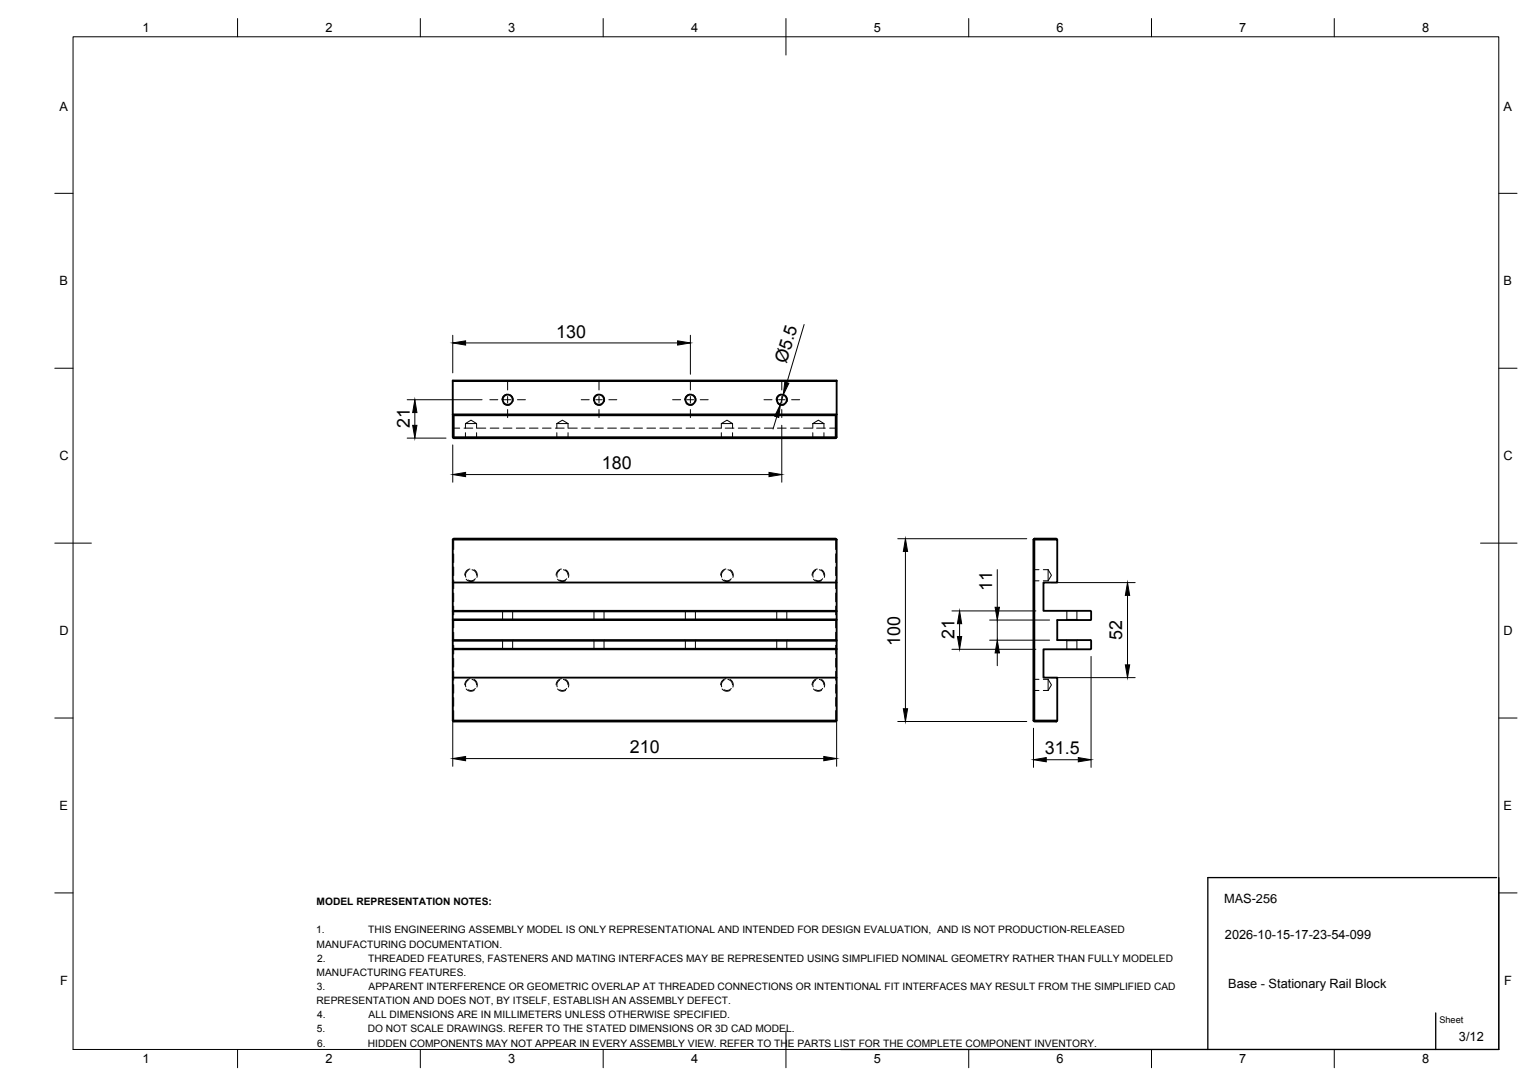
ISO-10303-21;
HEADER;
/* Generated by software containing ST-Developer
 * from STEP Tools, Inc. (www.steptools.com) 
 */

FILE_DESCRIPTION(
/* description */ (''),
/* implementation_level */ '2;1');

FILE_NAME(
/* name */ 'Base - Stationary Rail Block.step',
/* time_stamp */ '2026-10-14T18:40:07-07:00',
/* author */ (''),
/* organization */ (''),
/* preprocessor_version */ 'ST-DEVELOPER v20.2',
/* originating_system */ 'Autodesk Translation Framework v15.15.0.0',
/* authorisation */ '');

FILE_SCHEMA (('AUTOMOTIVE_DESIGN { 1 0 10303 214 3 1 1 }'));
ENDSEC;

DATA;
#10=MECHANICAL_DESIGN_GEOMETRIC_PRESENTATION_REPRESENTATION('',(#831),#81040);
#811=SHAPE_REPRESENTATION_RELATIONSHIP('SRR','None',#81130,#821);
#821=ADVANCED_BREP_SHAPE_REPRESENTATION('',(#841),#81030);
#831=STYLED_ITEM('',(#81189),#841);
#841=MANIFOLD_SOLID_BREP('Body1',#15084);
#851=CYLINDRICAL_SURFACE('',#15214,2.74999999999999);
#852=CYLINDRICAL_SURFACE('',#15218,2.75);
#853=CYLINDRICAL_SURFACE('',#15222,2.75);
#854=CYLINDRICAL_SURFACE('',#15226,2.75);
#855=CYLINDRICAL_SURFACE('',#15235,2.74999999999999);
#856=CYLINDRICAL_SURFACE('',#15239,2.75);
#857=CYLINDRICAL_SURFACE('',#15243,2.75);
#858=CYLINDRICAL_SURFACE('',#15247,2.75);
#859=CYLINDRICAL_SURFACE('',#15260,3.05);
#860=CYLINDRICAL_SURFACE('',#15264,3.05);
#861=CYLINDRICAL_SURFACE('',#15268,3.05);
#862=CYLINDRICAL_SURFACE('',#15272,3.05);
#863=CYLINDRICAL_SURFACE('',#15276,3.05);
#864=CYLINDRICAL_SURFACE('',#15280,3.05);
#865=CYLINDRICAL_SURFACE('',#15284,3.05);
#866=CYLINDRICAL_SURFACE('',#15288,3.05);
#1083=FACE_BOUND('',#2351,.T.);
#1084=FACE_BOUND('',#2352,.T.);
#1085=FACE_BOUND('',#2353,.T.);
#1086=FACE_BOUND('',#2354,.T.);
#1087=FACE_BOUND('',#2364,.T.);
#1088=FACE_BOUND('',#2365,.T.);
#1089=FACE_BOUND('',#2366,.T.);
#1090=FACE_BOUND('',#2367,.T.);
#1091=FACE_BOUND('',#2377,.T.);
#1092=FACE_BOUND('',#2378,.T.);
#1093=FACE_BOUND('',#2379,.T.);
#1094=FACE_BOUND('',#2380,.T.);
#1095=FACE_BOUND('',#2381,.T.);
#1096=FACE_BOUND('',#2382,.T.);
#1097=FACE_BOUND('',#2383,.T.);
#1098=FACE_BOUND('',#2384,.T.);
#1099=FACE_BOUND('',#2427,.T.);
#1100=FACE_BOUND('',#2428,.T.);
#1101=FACE_BOUND('',#2429,.T.);
#1102=FACE_BOUND('',#2430,.T.);
#1103=FACE_BOUND('',#2439,.T.);
#1104=FACE_BOUND('',#2440,.T.);
#1105=FACE_BOUND('',#2441,.T.);
#1106=FACE_BOUND('',#2442,.T.);
#1211=PLANE('',#15210);
#1212=PLANE('',#15231);
#1213=PLANE('',#15252);
#1214=PLANE('',#15298);
#1215=PLANE('',#15299);
#1216=PLANE('',#15300);
#1217=PLANE('',#15301);
#1218=PLANE('',#15302);
#1219=PLANE('',#15303);
#1220=PLANE('',#15304);
#1221=PLANE('',#15305);
#1222=PLANE('',#15306);
#1223=PLANE('',#15307);
#1224=PLANE('',#15308);
#1225=PLANE('',#15309);
#1226=PLANE('',#15310);
#1227=PLANE('',#15311);
#1228=PLANE('',#15312);
#1229=PLANE('',#15313);
#1230=PLANE('',#15314);
#1231=PLANE('',#15315);
#1232=PLANE('',#15316);
#1233=PLANE('',#15317);
#1234=PLANE('',#15318);
#1235=PLANE('',#15319);
#1236=PLANE('',#15320);
#1237=PLANE('',#15321);
#1238=PLANE('',#15322);
#1239=PLANE('',#15323);
#1240=PLANE('',#15324);
#1241=PLANE('',#15325);
#1242=PLANE('',#15326);
#1606=FACE_OUTER_BOUND('',#2349,.T.);
#1607=FACE_OUTER_BOUND('',#2350,.T.);
#1608=FACE_OUTER_BOUND('',#2355,.T.);
#1609=FACE_OUTER_BOUND('',#2356,.T.);
#1610=FACE_OUTER_BOUND('',#2357,.T.);
#1611=FACE_OUTER_BOUND('',#2358,.T.);
#1612=FACE_OUTER_BOUND('',#2359,.T.);
#1613=FACE_OUTER_BOUND('',#2360,.T.);
#1614=FACE_OUTER_BOUND('',#2361,.T.);
#1615=FACE_OUTER_BOUND('',#2362,.T.);
#1616=FACE_OUTER_BOUND('',#2363,.T.);
#1617=FACE_OUTER_BOUND('',#2368,.T.);
#1618=FACE_OUTER_BOUND('',#2369,.T.);
#1619=FACE_OUTER_BOUND('',#2370,.T.);
#1620=FACE_OUTER_BOUND('',#2371,.T.);
#1621=FACE_OUTER_BOUND('',#2372,.T.);
#1622=FACE_OUTER_BOUND('',#2373,.T.);
#1623=FACE_OUTER_BOUND('',#2374,.T.);
#1624=FACE_OUTER_BOUND('',#2375,.T.);
#1625=FACE_OUTER_BOUND('',#2376,.T.);
#1626=FACE_OUTER_BOUND('',#2385,.T.);
#1627=FACE_OUTER_BOUND('',#2386,.T.);
#1628=FACE_OUTER_BOUND('',#2387,.T.);
#1629=FACE_OUTER_BOUND('',#2388,.T.);
#1630=FACE_OUTER_BOUND('',#2389,.T.);
#1631=FACE_OUTER_BOUND('',#2390,.T.);
#1632=FACE_OUTER_BOUND('',#2391,.T.);
#1633=FACE_OUTER_BOUND('',#2392,.T.);
#1634=FACE_OUTER_BOUND('',#2393,.T.);
#1635=FACE_OUTER_BOUND('',#2394,.T.);
#1636=FACE_OUTER_BOUND('',#2395,.T.);
#1637=FACE_OUTER_BOUND('',#2396,.T.);
#1638=FACE_OUTER_BOUND('',#2397,.T.);
#1639=FACE_OUTER_BOUND('',#2398,.T.);
#1640=FACE_OUTER_BOUND('',#2399,.T.);
#1641=FACE_OUTER_BOUND('',#2400,.T.);
#1642=FACE_OUTER_BOUND('',#2401,.T.);
#1643=FACE_OUTER_BOUND('',#2402,.T.);
#1644=FACE_OUTER_BOUND('',#2403,.T.);
#1645=FACE_OUTER_BOUND('',#2404,.T.);
#1646=FACE_OUTER_BOUND('',#2405,.T.);
#1647=FACE_OUTER_BOUND('',#2406,.T.);
#1648=FACE_OUTER_BOUND('',#2407,.T.);
#1649=FACE_OUTER_BOUND('',#2408,.T.);
#1650=FACE_OUTER_BOUND('',#2409,.T.);
#1651=FACE_OUTER_BOUND('',#2410,.T.);
#1652=FACE_OUTER_BOUND('',#2411,.T.);
#1653=FACE_OUTER_BOUND('',#2412,.T.);
#1654=FACE_OUTER_BOUND('',#2413,.T.);
#1655=FACE_OUTER_BOUND('',#2414,.T.);
#1656=FACE_OUTER_BOUND('',#2415,.T.);
#1657=FACE_OUTER_BOUND('',#2416,.T.);
#1658=FACE_OUTER_BOUND('',#2417,.T.);
#1659=FACE_OUTER_BOUND('',#2418,.T.);
#1660=FACE_OUTER_BOUND('',#2419,.T.);
#1661=FACE_OUTER_BOUND('',#2420,.T.);
#1662=FACE_OUTER_BOUND('',#2421,.T.);
#1663=FACE_OUTER_BOUND('',#2422,.T.);
#1664=FACE_OUTER_BOUND('',#2423,.T.);
#1665=FACE_OUTER_BOUND('',#2424,.T.);
#1666=FACE_OUTER_BOUND('',#2425,.T.);
#1667=FACE_OUTER_BOUND('',#2426,.T.);
#1668=FACE_OUTER_BOUND('',#2431,.T.);
#1669=FACE_OUTER_BOUND('',#2432,.T.);
#1670=FACE_OUTER_BOUND('',#2433,.T.);
#1671=FACE_OUTER_BOUND('',#2434,.T.);
#1672=FACE_OUTER_BOUND('',#2435,.T.);
#1673=FACE_OUTER_BOUND('',#2436,.T.);
#1674=FACE_OUTER_BOUND('',#2437,.T.);
#1675=FACE_OUTER_BOUND('',#2438,.T.);
#1676=FACE_OUTER_BOUND('',#2443,.T.);
#1677=FACE_OUTER_BOUND('',#2444,.T.);
#2349=EDGE_LOOP('',(#9782,#9783,#9784,#9785));
#2350=EDGE_LOOP('',(#9786,#9787,#9788,#9789));
#2351=EDGE_LOOP('',(#9790));
#2352=EDGE_LOOP('',(#9791));
#2353=EDGE_LOOP('',(#9792));
#2354=EDGE_LOOP('',(#9793));
#2355=EDGE_LOOP('',(#9794,#9795,#9796,#9797));
#2356=EDGE_LOOP('',(#9798,#9799,#9800,#9801));
#2357=EDGE_LOOP('',(#9802,#9803,#9804,#9805));
#2358=EDGE_LOOP('',(#9806,#9807,#9808,#9809));
#2359=EDGE_LOOP('',(#9810,#9811,#9812,#9813));
#2360=EDGE_LOOP('',(#9814,#9815,#9816,#9817));
#2361=EDGE_LOOP('',(#9818,#9819,#9820,#9821));
#2362=EDGE_LOOP('',(#9822,#9823,#9824,#9825));
#2363=EDGE_LOOP('',(#9826,#9827,#9828,#9829));
#2364=EDGE_LOOP('',(#9830));
#2365=EDGE_LOOP('',(#9831));
#2366=EDGE_LOOP('',(#9832));
#2367=EDGE_LOOP('',(#9833));
#2368=EDGE_LOOP('',(#9834,#9835,#9836,#9837));
#2369=EDGE_LOOP('',(#9838,#9839,#9840,#9841));
#2370=EDGE_LOOP('',(#9842,#9843,#9844,#9845));
#2371=EDGE_LOOP('',(#9846,#9847,#9848,#9849));
#2372=EDGE_LOOP('',(#9850,#9851,#9852,#9853));
#2373=EDGE_LOOP('',(#9854,#9855,#9856,#9857));
#2374=EDGE_LOOP('',(#9858,#9859,#9860,#9861));
#2375=EDGE_LOOP('',(#9862,#9863,#9864,#9865));
#2376=EDGE_LOOP('',(#9866,#9867,#9868,#9869));
#2377=EDGE_LOOP('',(#9870));
#2378=EDGE_LOOP('',(#9871));
#2379=EDGE_LOOP('',(#9872));
#2380=EDGE_LOOP('',(#9873));
#2381=EDGE_LOOP('',(#9874));
#2382=EDGE_LOOP('',(#9875));
#2383=EDGE_LOOP('',(#9876));
#2384=EDGE_LOOP('',(#9877));
#2385=EDGE_LOOP('',(#9878,#9879,#9880,#9881));
#2386=EDGE_LOOP('',(#9882,#9883,#9884,#9885));
#2387=EDGE_LOOP('',(#9886,#9887,#9888,#9889));
#2388=EDGE_LOOP('',(#9890,#9891,#9892,#9893));
#2389=EDGE_LOOP('',(#9894,#9895,#9896,#9897));
#2390=EDGE_LOOP('',(#9898,#9899,#9900,#9901));
#2391=EDGE_LOOP('',(#9902,#9903,#9904,#9905));
#2392=EDGE_LOOP('',(#9906,#9907,#9908,#9909));
#2393=EDGE_LOOP('',(#9910,#9911,#9912,#9913));
#2394=EDGE_LOOP('',(#9914,#9915,#9916,#9917));
#2395=EDGE_LOOP('',(#9918,#9919,#9920,#9921));
#2396=EDGE_LOOP('',(#9922,#9923,#9924,#9925));
#2397=EDGE_LOOP('',(#9926,#9927,#9928,#9929));
#2398=EDGE_LOOP('',(#9930,#9931,#9932,#9933));
#2399=EDGE_LOOP('',(#9934,#9935,#9936,#9937));
#2400=EDGE_LOOP('',(#9938,#9939,#9940));
#2401=EDGE_LOOP('',(#9941,#9942,#9943));
#2402=EDGE_LOOP('',(#9944,#9945,#9946));
#2403=EDGE_LOOP('',(#9947,#9948,#9949));
#2404=EDGE_LOOP('',(#9950,#9951,#9952));
#2405=EDGE_LOOP('',(#9953,#9954,#9955));
#2406=EDGE_LOOP('',(#9956,#9957,#9958));
#2407=EDGE_LOOP('',(#9959,#9960,#9961));
#2408=EDGE_LOOP('',(#9962,#9963,#9964,#9965,#9966));
#2409=EDGE_LOOP('',(#9967,#9968,#9969,#9970,#9971,#9972));
#2410=EDGE_LOOP('',(#9973,#9974,#9975,#9976,#9977,#9978,#9979,#9980,#9981,
#9982,#9983,#9984,#9985,#9986,#9987,#9988,#9989,#9990,#9991,#9992));
#2411=EDGE_LOOP('',(#9993,#9994,#9995,#9996));
#2412=EDGE_LOOP('',(#9997,#9998,#9999,#10000,#10001,#10002));
#2413=EDGE_LOOP('',(#10003,#10004,#10005,#10006,#10007));
#2414=EDGE_LOOP('',(#10008,#10009,#10010,#10011));
#2415=EDGE_LOOP('',(#10012,#10013,#10014,#10015,#10016));
#2416=EDGE_LOOP('',(#10017,#10018,#10019,#10020,#10021,#10022));
#2417=EDGE_LOOP('',(#10023,#10024,#10025,#10026,#10027,#10028));
#2418=EDGE_LOOP('',(#10029,#10030,#10031,#10032,#10033));
#2419=EDGE_LOOP('',(#10034,#10035,#10036,#10037,#10038,#10039,#10040,#10041,
#10042,#10043,#10044,#10045,#10046,#10047,#10048,#10049,#10050,#10051,#10052,
#10053));
#2420=EDGE_LOOP('',(#10054,#10055,#10056,#10057));
#2421=EDGE_LOOP('',(#10058,#10059,#10060,#10061));
#2422=EDGE_LOOP('',(#10062,#10063,#10064,#10065));
#2423=EDGE_LOOP('',(#10066,#10067,#10068,#10069));
#2424=EDGE_LOOP('',(#10070,#10071,#10072,#10073));
#2425=EDGE_LOOP('',(#10074,#10075,#10076,#10077));
#2426=EDGE_LOOP('',(#10078,#10079,#10080,#10081));
#2427=EDGE_LOOP('',(#10082));
#2428=EDGE_LOOP('',(#10083));
#2429=EDGE_LOOP('',(#10084));
#2430=EDGE_LOOP('',(#10085));
#2431=EDGE_LOOP('',(#10086,#10087,#10088,#10089));
#2432=EDGE_LOOP('',(#10090,#10091,#10092,#10093));
#2433=EDGE_LOOP('',(#10094,#10095,#10096,#10097));
#2434=EDGE_LOOP('',(#10098,#10099,#10100,#10101));
#2435=EDGE_LOOP('',(#10102,#10103,#10104,#10105));
#2436=EDGE_LOOP('',(#10106,#10107,#10108,#10109));
#2437=EDGE_LOOP('',(#10110,#10111,#10112,#10113));
#2438=EDGE_LOOP('',(#10114,#10115,#10116,#10117));
#2439=EDGE_LOOP('',(#10118));
#2440=EDGE_LOOP('',(#10119));
#2441=EDGE_LOOP('',(#10120));
#2442=EDGE_LOOP('',(#10121));
#2443=EDGE_LOOP('',(#10122,#10123,#10124,#10125));
#2444=EDGE_LOOP('',(#10126,#10127,#10128,#10129));
#3220=LINE('',#20568,#4332);
#3221=LINE('',#20573,#4333);
#3222=LINE('',#20575,#4334);
#3223=LINE('',#20577,#4335);
#3224=LINE('',#20578,#4336);
#3225=LINE('',#20587,#4337);
#3226=LINE('',#20592,#4338);
#3227=LINE('',#20595,#4339);
#3228=LINE('',#20600,#4340);
#3229=LINE('',#20603,#4341);
#3230=LINE('',#20608,#4342);
#3231=LINE('',#20611,#4343);
#3232=LINE('',#20617,#4344);
#3233=LINE('',#20622,#4345);
#3234=LINE('',#20624,#4346);
#3235=LINE('',#20626,#4347);
#3236=LINE('',#20627,#4348);
#3237=LINE('',#20636,#4349);
#3238=LINE('',#20641,#4350);
#3239=LINE('',#20644,#4351);
#3240=LINE('',#20649,#4352);
#3241=LINE('',#20652,#4353);
#3242=LINE('',#20657,#4354);
#3243=LINE('',#20660,#4355);
#3244=LINE('',#20666,#4356);
#3245=LINE('',#20671,#4357);
#3246=LINE('',#20673,#4358);
#3247=LINE('',#20675,#4359);
#3248=LINE('',#20676,#4360);
#3249=LINE('',#20693,#4361);
#3250=LINE('',#20698,#4362);
#3251=LINE('',#20701,#4363);
#3252=LINE('',#20706,#4364);
#3253=LINE('',#20709,#4365);
#3254=LINE('',#20714,#4366);
#3255=LINE('',#20717,#4367);
#3256=LINE('',#20722,#4368);
#3257=LINE('',#20725,#4369);
#3258=LINE('',#20730,#4370);
#3259=LINE('',#20733,#4371);
#3260=LINE('',#20738,#4372);
#3261=LINE('',#20741,#4373);
#3262=LINE('',#20746,#4374);
#3263=LINE('',#20749,#4375);
#3264=LINE('',#20753,#4376);
#3265=LINE('',#20756,#4377);
#3266=LINE('',#20759,#4378);
#3267=LINE('',#20762,#4379);
#3268=LINE('',#20765,#4380);
#3269=LINE('',#20768,#4381);
#3270=LINE('',#20771,#4382);
#3271=LINE('',#20774,#4383);
#3272=LINE('',#20778,#4384);
#3273=LINE('',#20780,#4385);
#3274=LINE('',#20782,#4386);
#3275=LINE('',#20784,#4387);
#3276=LINE('',#20785,#4388);
#3277=LINE('',#20788,#4389);
#3278=LINE('',#20790,#4390);
#3279=LINE('',#20791,#4391);
#3280=LINE('',#20792,#4392);
#3281=LINE('',#20795,#4393);
#3282=LINE('',#20797,#4394);
#3283=LINE('',#20799,#4395);
#3284=LINE('',#20801,#4396);
#3285=LINE('',#20803,#4397);
#3286=LINE('',#20805,#4398);
#3287=LINE('',#20806,#4399);
#3288=LINE('',#20807,#4400);
#3289=LINE('',#20809,#4401);
#3290=LINE('',#20811,#4402);
#3291=LINE('',#20813,#4403);
#3292=LINE('',#20815,#4404);
#3293=LINE('',#20817,#4405);
#3294=LINE('',#20819,#4406);
#3295=LINE('',#20821,#4407);
#3296=LINE('',#20822,#4408);
#3297=LINE('',#20825,#4409);
#3298=LINE('',#20827,#4410);
#3299=LINE('',#20828,#4411);
#3300=LINE('',#20831,#4412);
#3301=LINE('',#20833,#4413);
#3302=LINE('',#20835,#4414);
#3303=LINE('',#20836,#4415);
#3304=LINE('',#20839,#4416);
#3305=LINE('',#20840,#4417);
#3306=LINE('',#20843,#4418);
#3307=LINE('',#20844,#4419);
#3308=LINE('',#20847,#4420);
#3309=LINE('',#20849,#4421);
#3310=LINE('',#20850,#4422);
#3311=LINE('',#20853,#4423);
#3312=LINE('',#20855,#4424);
#3313=LINE('',#20856,#4425);
#3314=LINE('',#20859,#4426);
#3315=LINE('',#20860,#4427);
#3316=LINE('',#20862,#4428);
#3317=LINE('',#20863,#4429);
#3318=LINE('',#20866,#4430);
#3319=LINE('',#20868,#4431);
#3320=LINE('',#20870,#4432);
#3321=LINE('',#20872,#4433);
#3322=LINE('',#20874,#4434);
#3323=LINE('',#20876,#4435);
#3324=LINE('',#20877,#4436);
#3325=LINE('',#20878,#4437);
#3326=LINE('',#20880,#4438);
#3327=LINE('',#20882,#4439);
#3328=LINE('',#20884,#4440);
#3329=LINE('',#20886,#4441);
#3330=LINE('',#20888,#4442);
#3331=LINE('',#20890,#4443);
#3332=LINE('',#20891,#4444);
#3333=LINE('',#20893,#4445);
#3334=LINE('',#20894,#4446);
#3335=LINE('',#20896,#4447);
#3336=LINE('',#20899,#4448);
#3337=LINE('',#20901,#4449);
#3338=LINE('',#20903,#4450);
#3339=LINE('',#20905,#4451);
#3340=LINE('',#20907,#4452);
#3341=LINE('',#20909,#4453);
#3342=LINE('',#20912,#4454);
#3343=LINE('',#20914,#4455);
#3344=LINE('',#20918,#4456);
#3345=LINE('',#20920,#4457);
#4332=VECTOR('',#16628,2.89999999999999);
#4333=VECTOR('',#16633,10.);
#4334=VECTOR('',#16634,10.);
#4335=VECTOR('',#16635,10.);
#4336=VECTOR('',#16636,10.);
#4337=VECTOR('',#16645,2.74999999999999);
#4338=VECTOR('',#16652,2.9);
#4339=VECTOR('',#16655,2.75);
#4340=VECTOR('',#16662,2.9);
#4341=VECTOR('',#16665,2.75);
#4342=VECTOR('',#16672,2.9);
#4343=VECTOR('',#16675,2.75);
#4344=VECTOR('',#16682,2.89999999999999);
#4345=VECTOR('',#16687,10.);
#4346=VECTOR('',#16688,10.);
#4347=VECTOR('',#16689,10.);
#4348=VECTOR('',#16690,10.);
#4349=VECTOR('',#16699,2.74999999999999);
#4350=VECTOR('',#16706,2.9);
#4351=VECTOR('',#16709,2.75);
#4352=VECTOR('',#16716,2.9);
#4353=VECTOR('',#16719,2.75);
#4354=VECTOR('',#16726,2.9);
#4355=VECTOR('',#16729,2.75);
#4356=VECTOR('',#16736,3.24999999999999);
#4357=VECTOR('',#16741,10.);
#4358=VECTOR('',#16742,10.);
#4359=VECTOR('',#16743,10.);
#4360=VECTOR('',#16744,10.);
#4361=VECTOR('',#16761,3.05);
#4362=VECTOR('',#16768,3.24999999999999);
#4363=VECTOR('',#16771,3.05);
#4364=VECTOR('',#16778,3.25);
#4365=VECTOR('',#16781,3.05);
#4366=VECTOR('',#16788,3.25);
#4367=VECTOR('',#16791,3.05);
#4368=VECTOR('',#16798,3.25);
#4369=VECTOR('',#16801,3.05);
#4370=VECTOR('',#16808,3.25);
#4371=VECTOR('',#16811,3.05);
#4372=VECTOR('',#16818,3.24999999999999);
#4373=VECTOR('',#16821,3.05);
#4374=VECTOR('',#16828,3.24999999999999);
#4375=VECTOR('',#16831,3.05);
#4376=VECTOR('',#16836,1.525);
#4377=VECTOR('',#16839,1.525);
#4378=VECTOR('',#16842,1.525);
#4379=VECTOR('',#16845,1.525);
#4380=VECTOR('',#16848,1.525);
#4381=VECTOR('',#16851,1.525);
#4382=VECTOR('',#16854,1.525);
#4383=VECTOR('',#16857,1.525);
#4384=VECTOR('',#16860,10.);
#4385=VECTOR('',#16861,10.);
#4386=VECTOR('',#16862,10.);
#4387=VECTOR('',#16863,10.);
#4388=VECTOR('',#16864,10.);
#4389=VECTOR('',#16867,10.);
#4390=VECTOR('',#16868,10.);
#4391=VECTOR('',#16869,10.);
#4392=VECTOR('',#16870,10.);
#4393=VECTOR('',#16873,10.);
#4394=VECTOR('',#16874,10.);
#4395=VECTOR('',#16875,10.);
#4396=VECTOR('',#16876,10.);
#4397=VECTOR('',#16877,10.);
#4398=VECTOR('',#16878,10.);
#4399=VECTOR('',#16879,10.);
#4400=VECTOR('',#16880,10.);
#4401=VECTOR('',#16881,10.);
#4402=VECTOR('',#16882,10.);
#4403=VECTOR('',#16883,10.);
#4404=VECTOR('',#16884,10.);
#4405=VECTOR('',#16885,10.);
#4406=VECTOR('',#16886,10.);
#4407=VECTOR('',#16887,10.);
#4408=VECTOR('',#16888,10.);
#4409=VECTOR('',#16891,10.);
#4410=VECTOR('',#16892,10.);
#4411=VECTOR('',#16893,10.);
#4412=VECTOR('',#16896,10.);
#4413=VECTOR('',#16897,10.);
#4414=VECTOR('',#16898,10.);
#4415=VECTOR('',#16899,10.);
#4416=VECTOR('',#16902,10.);
#4417=VECTOR('',#16903,10.);
#4418=VECTOR('',#16906,10.);
#4419=VECTOR('',#16907,10.);
#4420=VECTOR('',#16910,10.);
#4421=VECTOR('',#16911,10.);
#4422=VECTOR('',#16912,10.);
#4423=VECTOR('',#16915,10.);
#4424=VECTOR('',#16916,10.);
#4425=VECTOR('',#16917,10.);
#4426=VECTOR('',#16920,10.);
#4427=VECTOR('',#16921,10.);
#4428=VECTOR('',#16924,10.);
#4429=VECTOR('',#16925,10.);
#4430=VECTOR('',#16928,10.);
#4431=VECTOR('',#16929,10.);
#4432=VECTOR('',#16930,10.);
#4433=VECTOR('',#16931,10.);
#4434=VECTOR('',#16932,10.);
#4435=VECTOR('',#16933,10.);
#4436=VECTOR('',#16934,10.);
#4437=VECTOR('',#16935,10.);
#4438=VECTOR('',#16936,10.);
#4439=VECTOR('',#16937,10.);
#4440=VECTOR('',#16938,10.);
#4441=VECTOR('',#16939,10.);
#4442=VECTOR('',#16940,10.);
#4443=VECTOR('',#16941,10.);
#4444=VECTOR('',#16942,10.);
#4445=VECTOR('',#16945,10.);
#4446=VECTOR('',#16946,10.);
#4447=VECTOR('',#16949,10.);
#4448=VECTOR('',#16954,10.);
#4449=VECTOR('',#16957,10.);
#4450=VECTOR('',#16960,10.);
#4451=VECTOR('',#16963,10.);
#4452=VECTOR('',#16966,10.);
#4453=VECTOR('',#16969,10.);
#4454=VECTOR('',#16974,10.);
#4455=VECTOR('',#16977,10.);
#4456=VECTOR('',#16984,10.);
#4457=VECTOR('',#16987,10.);
#5444=CIRCLE('',#15208,2.74999999999999);
#5445=CIRCLE('',#15209,3.05);
#5446=CIRCLE('',#15211,3.05);
#5447=CIRCLE('',#15212,3.05);
#5448=CIRCLE('',#15213,3.05);
#5449=CIRCLE('',#15215,2.74999999999999);
#5450=CIRCLE('',#15217,2.75);
#5451=CIRCLE('',#15219,2.75);
#5452=CIRCLE('',#15221,2.75);
#5453=CIRCLE('',#15223,2.75);
#5454=CIRCLE('',#15225,2.75);
#5455=CIRCLE('',#15227,2.75);
#5456=CIRCLE('',#15229,2.74999999999999);
#5457=CIRCLE('',#15230,3.05);
#5458=CIRCLE('',#15232,3.05);
#5459=CIRCLE('',#15233,3.05);
#5460=CIRCLE('',#15234,3.05);
#5461=CIRCLE('',#15236,2.74999999999999);
#5462=CIRCLE('',#15238,2.75);
#5463=CIRCLE('',#15240,2.75);
#5464=CIRCLE('',#15242,2.75);
#5465=CIRCLE('',#15244,2.75);
#5466=CIRCLE('',#15246,2.75);
#5467=CIRCLE('',#15248,2.75);
#5468=CIRCLE('',#15250,3.05);
#5469=CIRCLE('',#15251,3.44999999999999);
#5470=CIRCLE('',#15253,3.44999999999999);
#5471=CIRCLE('',#15254,3.45);
#5472=CIRCLE('',#15255,3.45);
#5473=CIRCLE('',#15256,3.44999999999999);
#5474=CIRCLE('',#15257,3.44999999999999);
#5475=CIRCLE('',#15258,3.45);
#5476=CIRCLE('',#15259,3.45);
#5477=CIRCLE('',#15261,3.05);
#5478=CIRCLE('',#15263,3.05);
#5479=CIRCLE('',#15265,3.05);
#5480=CIRCLE('',#15267,3.05);
#5481=CIRCLE('',#15269,3.05);
#5482=CIRCLE('',#15271,3.05);
#5483=CIRCLE('',#15273,3.05);
#5484=CIRCLE('',#15275,3.05);
#5485=CIRCLE('',#15277,3.05);
#5486=CIRCLE('',#15279,3.05);
#5487=CIRCLE('',#15281,3.05);
#5488=CIRCLE('',#15283,3.05);
#5489=CIRCLE('',#15285,3.05);
#5490=CIRCLE('',#15287,3.05);
#5491=CIRCLE('',#15289,3.05);
#6021=VERTEX_POINT('',#20565);
#6022=VERTEX_POINT('',#20567);
#6023=VERTEX_POINT('',#20571);
#6024=VERTEX_POINT('',#20572);
#6025=VERTEX_POINT('',#20574);
#6026=VERTEX_POINT('',#20576);
#6027=VERTEX_POINT('',#20579);
#6028=VERTEX_POINT('',#20581);
#6029=VERTEX_POINT('',#20583);
#6030=VERTEX_POINT('',#20586);
#6031=VERTEX_POINT('',#20590);
#6032=VERTEX_POINT('',#20594);
#6033=VERTEX_POINT('',#20598);
#6034=VERTEX_POINT('',#20602);
#6035=VERTEX_POINT('',#20606);
#6036=VERTEX_POINT('',#20610);
#6037=VERTEX_POINT('',#20614);
#6038=VERTEX_POINT('',#20616);
#6039=VERTEX_POINT('',#20620);
#6040=VERTEX_POINT('',#20621);
#6041=VERTEX_POINT('',#20623);
#6042=VERTEX_POINT('',#20625);
#6043=VERTEX_POINT('',#20628);
#6044=VERTEX_POINT('',#20630);
#6045=VERTEX_POINT('',#20632);
#6046=VERTEX_POINT('',#20635);
#6047=VERTEX_POINT('',#20639);
#6048=VERTEX_POINT('',#20643);
#6049=VERTEX_POINT('',#20647);
#6050=VERTEX_POINT('',#20651);
#6051=VERTEX_POINT('',#20655);
#6052=VERTEX_POINT('',#20659);
#6053=VERTEX_POINT('',#20663);
#6054=VERTEX_POINT('',#20665);
#6055=VERTEX_POINT('',#20669);
#6056=VERTEX_POINT('',#20670);
#6057=VERTEX_POINT('',#20672);
#6058=VERTEX_POINT('',#20674);
#6059=VERTEX_POINT('',#20677);
#6060=VERTEX_POINT('',#20679);
#6061=VERTEX_POINT('',#20681);
#6062=VERTEX_POINT('',#20683);
#6063=VERTEX_POINT('',#20685);
#6064=VERTEX_POINT('',#20687);
#6065=VERTEX_POINT('',#20689);
#6066=VERTEX_POINT('',#20692);
#6067=VERTEX_POINT('',#20696);
#6068=VERTEX_POINT('',#20700);
#6069=VERTEX_POINT('',#20704);
#6070=VERTEX_POINT('',#20708);
#6071=VERTEX_POINT('',#20712);
#6072=VERTEX_POINT('',#20716);
#6073=VERTEX_POINT('',#20720);
#6074=VERTEX_POINT('',#20724);
#6075=VERTEX_POINT('',#20728);
#6076=VERTEX_POINT('',#20732);
#6077=VERTEX_POINT('',#20736);
#6078=VERTEX_POINT('',#20740);
#6079=VERTEX_POINT('',#20744);
#6080=VERTEX_POINT('',#20748);
#6081=VERTEX_POINT('',#20752);
#6082=VERTEX_POINT('',#20755);
#6083=VERTEX_POINT('',#20758);
#6084=VERTEX_POINT('',#20761);
#6085=VERTEX_POINT('',#20764);
#6086=VERTEX_POINT('',#20767);
#6087=VERTEX_POINT('',#20770);
#6088=VERTEX_POINT('',#20773);
#6089=VERTEX_POINT('',#20776);
#6090=VERTEX_POINT('',#20777);
#6091=VERTEX_POINT('',#20779);
#6092=VERTEX_POINT('',#20781);
#6093=VERTEX_POINT('',#20783);
#6094=VERTEX_POINT('',#20787);
#6095=VERTEX_POINT('',#20789);
#6096=VERTEX_POINT('',#20794);
#6097=VERTEX_POINT('',#20796);
#6098=VERTEX_POINT('',#20798);
#6099=VERTEX_POINT('',#20800);
#6100=VERTEX_POINT('',#20802);
#6101=VERTEX_POINT('',#20804);
#6102=VERTEX_POINT('',#20808);
#6103=VERTEX_POINT('',#20810);
#6104=VERTEX_POINT('',#20812);
#6105=VERTEX_POINT('',#20814);
#6106=VERTEX_POINT('',#20816);
#6107=VERTEX_POINT('',#20818);
#6108=VERTEX_POINT('',#20820);
#6109=VERTEX_POINT('',#20824);
#6110=VERTEX_POINT('',#20826);
#6111=VERTEX_POINT('',#20830);
#6112=VERTEX_POINT('',#20832);
#6113=VERTEX_POINT('',#20834);
#6114=VERTEX_POINT('',#20838);
#6115=VERTEX_POINT('',#20842);
#6116=VERTEX_POINT('',#20846);
#6117=VERTEX_POINT('',#20848);
#6118=VERTEX_POINT('',#20852);
#6119=VERTEX_POINT('',#20854);
#6120=VERTEX_POINT('',#20858);
#6121=VERTEX_POINT('',#20865);
#6122=VERTEX_POINT('',#20867);
#6123=VERTEX_POINT('',#20869);
#6124=VERTEX_POINT('',#20871);
#6125=VERTEX_POINT('',#20873);
#6126=VERTEX_POINT('',#20875);
#6127=VERTEX_POINT('',#20879);
#6128=VERTEX_POINT('',#20881);
#6129=VERTEX_POINT('',#20883);
#6130=VERTEX_POINT('',#20885);
#6131=VERTEX_POINT('',#20887);
#6132=VERTEX_POINT('',#20889);
#7554=EDGE_CURVE('',#6021,#6021,#5444,.T.);
#7555=EDGE_CURVE('',#6021,#6022,#3220,.T.);
#7556=EDGE_CURVE('',#6022,#6022,#5445,.T.);
#7557=EDGE_CURVE('',#6023,#6024,#3221,.T.);
#7558=EDGE_CURVE('',#6025,#6023,#3222,.T.);
#7559=EDGE_CURVE('',#6026,#6025,#3223,.T.);
#7560=EDGE_CURVE('',#6024,#6026,#3224,.T.);
#7561=EDGE_CURVE('',#6027,#6027,#5446,.T.);
#7562=EDGE_CURVE('',#6028,#6028,#5447,.T.);
#7563=EDGE_CURVE('',#6029,#6029,#5448,.T.);
#7564=EDGE_CURVE('',#6021,#6030,#3225,.T.);
#7565=EDGE_CURVE('',#6030,#6030,#5449,.T.);
#7566=EDGE_CURVE('',#6031,#6031,#5450,.T.);
#7567=EDGE_CURVE('',#6031,#6027,#3226,.T.);
#7568=EDGE_CURVE('',#6031,#6032,#3227,.T.);
#7569=EDGE_CURVE('',#6032,#6032,#5451,.T.);
#7570=EDGE_CURVE('',#6033,#6033,#5452,.T.);
#7571=EDGE_CURVE('',#6033,#6029,#3228,.T.);
#7572=EDGE_CURVE('',#6033,#6034,#3229,.T.);
#7573=EDGE_CURVE('',#6034,#6034,#5453,.T.);
#7574=EDGE_CURVE('',#6035,#6035,#5454,.T.);
#7575=EDGE_CURVE('',#6035,#6028,#3230,.T.);
#7576=EDGE_CURVE('',#6035,#6036,#3231,.T.);
#7577=EDGE_CURVE('',#6036,#6036,#5455,.T.);
#7578=EDGE_CURVE('',#6037,#6037,#5456,.T.);
#7579=EDGE_CURVE('',#6037,#6038,#3232,.T.);
#7580=EDGE_CURVE('',#6038,#6038,#5457,.T.);
#7581=EDGE_CURVE('',#6039,#6040,#3233,.T.);
#7582=EDGE_CURVE('',#6041,#6039,#3234,.T.);
#7583=EDGE_CURVE('',#6041,#6042,#3235,.T.);
#7584=EDGE_CURVE('',#6040,#6042,#3236,.T.);
#7585=EDGE_CURVE('',#6043,#6043,#5458,.T.);
#7586=EDGE_CURVE('',#6044,#6044,#5459,.T.);
#7587=EDGE_CURVE('',#6045,#6045,#5460,.T.);
#7588=EDGE_CURVE('',#6037,#6046,#3237,.T.);
#7589=EDGE_CURVE('',#6046,#6046,#5461,.T.);
#7590=EDGE_CURVE('',#6047,#6047,#5462,.T.);
#7591=EDGE_CURVE('',#6047,#6043,#3238,.T.);
#7592=EDGE_CURVE('',#6047,#6048,#3239,.T.);
#7593=EDGE_CURVE('',#6048,#6048,#5463,.T.);
#7594=EDGE_CURVE('',#6049,#6049,#5464,.T.);
#7595=EDGE_CURVE('',#6049,#6045,#3240,.T.);
#7596=EDGE_CURVE('',#6049,#6050,#3241,.T.);
#7597=EDGE_CURVE('',#6050,#6050,#5465,.T.);
#7598=EDGE_CURVE('',#6051,#6051,#5466,.T.);
#7599=EDGE_CURVE('',#6051,#6044,#3242,.T.);
#7600=EDGE_CURVE('',#6051,#6052,#3243,.T.);
#7601=EDGE_CURVE('',#6052,#6052,#5467,.T.);
#7602=EDGE_CURVE('',#6053,#6053,#5468,.T.);
#7603=EDGE_CURVE('',#6053,#6054,#3244,.T.);
#7604=EDGE_CURVE('',#6054,#6054,#5469,.T.);
#7605=EDGE_CURVE('',#6055,#6056,#3245,.T.);
#7606=EDGE_CURVE('',#6057,#6055,#3246,.T.);
#7607=EDGE_CURVE('',#6058,#6057,#3247,.T.);
#7608=EDGE_CURVE('',#6056,#6058,#3248,.T.);
#7609=EDGE_CURVE('',#6059,#6059,#5470,.T.);
#7610=EDGE_CURVE('',#6060,#6060,#5471,.T.);
#7611=EDGE_CURVE('',#6061,#6061,#5472,.T.);
#7612=EDGE_CURVE('',#6062,#6062,#5473,.T.);
#7613=EDGE_CURVE('',#6063,#6063,#5474,.T.);
#7614=EDGE_CURVE('',#6064,#6064,#5475,.T.);
#7615=EDGE_CURVE('',#6065,#6065,#5476,.T.);
#7616=EDGE_CURVE('',#6053,#6066,#3249,.T.);
#7617=EDGE_CURVE('',#6066,#6066,#5477,.T.);
#7618=EDGE_CURVE('',#6067,#6067,#5478,.T.);
#7619=EDGE_CURVE('',#6067,#6059,#3250,.T.);
#7620=EDGE_CURVE('',#6067,#6068,#3251,.T.);
#7621=EDGE_CURVE('',#6068,#6068,#5479,.T.);
#7622=EDGE_CURVE('',#6069,#6069,#5480,.T.);
#7623=EDGE_CURVE('',#6069,#6065,#3252,.T.);
#7624=EDGE_CURVE('',#6069,#6070,#3253,.T.);
#7625=EDGE_CURVE('',#6070,#6070,#5481,.T.);
#7626=EDGE_CURVE('',#6071,#6071,#5482,.T.);
#7627=EDGE_CURVE('',#6071,#6060,#3254,.T.);
#7628=EDGE_CURVE('',#6071,#6072,#3255,.T.);
#7629=EDGE_CURVE('',#6072,#6072,#5483,.T.);
#7630=EDGE_CURVE('',#6073,#6073,#5484,.T.);
#7631=EDGE_CURVE('',#6073,#6064,#3256,.T.);
#7632=EDGE_CURVE('',#6073,#6074,#3257,.T.);
#7633=EDGE_CURVE('',#6074,#6074,#5485,.T.);
#7634=EDGE_CURVE('',#6075,#6075,#5486,.T.);
#7635=EDGE_CURVE('',#6075,#6061,#3258,.T.);
#7636=EDGE_CURVE('',#6075,#6076,#3259,.T.);
#7637=EDGE_CURVE('',#6076,#6076,#5487,.T.);
#7638=EDGE_CURVE('',#6077,#6077,#5488,.T.);
#7639=EDGE_CURVE('',#6077,#6063,#3260,.T.);
#7640=EDGE_CURVE('',#6077,#6078,#3261,.T.);
#7641=EDGE_CURVE('',#6078,#6078,#5489,.T.);
#7642=EDGE_CURVE('',#6079,#6079,#5490,.T.);
#7643=EDGE_CURVE('',#6079,#6062,#3262,.T.);
#7644=EDGE_CURVE('',#6079,#6080,#3263,.T.);
#7645=EDGE_CURVE('',#6080,#6080,#5491,.T.);
#7646=EDGE_CURVE('',#6081,#6066,#3264,.T.);
#7647=EDGE_CURVE('',#6082,#6080,#3265,.T.);
#7648=EDGE_CURVE('',#6083,#6068,#3266,.T.);
#7649=EDGE_CURVE('',#6084,#6078,#3267,.T.);
#7650=EDGE_CURVE('',#6085,#6076,#3268,.T.);
#7651=EDGE_CURVE('',#6086,#6072,#3269,.T.);
#7652=EDGE_CURVE('',#6087,#6074,#3270,.T.);
#7653=EDGE_CURVE('',#6088,#6070,#3271,.T.);
#7654=EDGE_CURVE('',#6089,#6090,#3272,.T.);
#7655=EDGE_CURVE('',#6090,#6091,#3273,.T.);
#7656=EDGE_CURVE('',#6091,#6092,#3274,.T.);
#7657=EDGE_CURVE('',#6092,#6093,#3275,.T.);
#7658=EDGE_CURVE('',#6093,#6089,#3276,.T.);
#7659=EDGE_CURVE('',#6091,#6094,#3277,.T.);
#7660=EDGE_CURVE('',#6094,#6095,#3278,.T.);
#7661=EDGE_CURVE('',#6095,#6055,#3279,.T.);
#7662=EDGE_CURVE('',#6056,#6092,#3280,.T.);
#7663=EDGE_CURVE('',#6090,#6096,#3281,.T.);
#7664=EDGE_CURVE('',#6096,#6097,#3282,.T.);
#7665=EDGE_CURVE('',#6097,#6098,#3283,.T.);
#7666=EDGE_CURVE('',#6098,#6099,#3284,.T.);
#7667=EDGE_CURVE('',#6100,#6099,#3285,.T.);
#7668=EDGE_CURVE('',#6100,#6101,#3286,.T.);
#7669=EDGE_CURVE('',#6040,#6101,#3287,.T.);
#7670=EDGE_CURVE('',#6042,#6025,#3288,.T.);
#7671=EDGE_CURVE('',#6102,#6023,#3289,.T.);
#7672=EDGE_CURVE('',#6102,#6103,#3290,.T.);
#7673=EDGE_CURVE('',#6104,#6103,#3291,.T.);
#7674=EDGE_CURVE('',#6104,#6105,#3292,.T.);
#7675=EDGE_CURVE('',#6105,#6106,#3293,.T.);
#7676=EDGE_CURVE('',#6106,#6107,#3294,.T.);
#7677=EDGE_CURVE('',#6107,#6108,#3295,.T.);
#7678=EDGE_CURVE('',#6094,#6108,#3296,.T.);
#7679=EDGE_CURVE('',#6089,#6109,#3297,.T.);
#7680=EDGE_CURVE('',#6110,#6109,#3298,.T.);
#7681=EDGE_CURVE('',#6110,#6090,#3299,.T.);
#7682=EDGE_CURVE('',#6111,#6095,#3300,.T.);
#7683=EDGE_CURVE('',#6111,#6112,#3301,.T.);
#7684=EDGE_CURVE('',#6113,#6112,#3302,.T.);
#7685=EDGE_CURVE('',#6057,#6113,#3303,.T.);
#7686=EDGE_CURVE('',#6108,#6114,#3304,.T.);
#7687=EDGE_CURVE('',#6114,#6111,#3305,.T.);
#7688=EDGE_CURVE('',#6115,#6114,#3306,.T.);
#7689=EDGE_CURVE('',#6112,#6115,#3307,.T.);
#7690=EDGE_CURVE('',#6115,#6116,#3308,.T.);
#7691=EDGE_CURVE('',#6116,#6117,#3309,.T.);
#7692=EDGE_CURVE('',#6117,#6113,#3310,.T.);
#7693=EDGE_CURVE('',#6117,#6118,#3311,.T.);
#7694=EDGE_CURVE('',#6118,#6119,#3312,.T.);
#7695=EDGE_CURVE('',#6119,#6058,#3313,.T.);
#7696=EDGE_CURVE('',#6120,#6119,#3314,.T.);
#7697=EDGE_CURVE('',#6120,#6093,#3315,.T.);
#7698=EDGE_CURVE('',#6118,#6110,#3316,.T.);
#7699=EDGE_CURVE('',#6109,#6120,#3317,.T.);
#7700=EDGE_CURVE('',#6116,#6121,#3318,.T.);
#7701=EDGE_CURVE('',#6121,#6122,#3319,.T.);
#7702=EDGE_CURVE('',#6122,#6123,#3320,.T.);
#7703=EDGE_CURVE('',#6123,#6124,#3321,.T.);
#7704=EDGE_CURVE('',#6125,#6124,#3322,.T.);
#7705=EDGE_CURVE('',#6125,#6126,#3323,.T.);
#7706=EDGE_CURVE('',#6024,#6126,#3324,.T.);
#7707=EDGE_CURVE('',#6026,#6041,#3325,.T.);
#7708=EDGE_CURVE('',#6127,#6039,#3326,.T.);
#7709=EDGE_CURVE('',#6127,#6128,#3327,.T.);
#7710=EDGE_CURVE('',#6129,#6128,#3328,.T.);
#7711=EDGE_CURVE('',#6129,#6130,#3329,.T.);
#7712=EDGE_CURVE('',#6130,#6131,#3330,.T.);
#7713=EDGE_CURVE('',#6131,#6132,#3331,.T.);
#7714=EDGE_CURVE('',#6132,#6110,#3332,.T.);
#7715=EDGE_CURVE('',#6099,#6129,#3333,.T.);
#7716=EDGE_CURVE('',#6128,#6100,#3334,.T.);
#7717=EDGE_CURVE('',#6101,#6127,#3335,.T.);
#7718=EDGE_CURVE('',#6126,#6102,#3336,.T.);
#7719=EDGE_CURVE('',#6103,#6125,#3337,.T.);
#7720=EDGE_CURVE('',#6124,#6104,#3338,.T.);
#7721=EDGE_CURVE('',#6123,#6105,#3339,.T.);
#7722=EDGE_CURVE('',#6108,#6116,#3340,.T.);
#7723=EDGE_CURVE('',#6132,#6096,#3341,.T.);
#7724=EDGE_CURVE('',#6121,#6107,#3342,.T.);
#7725=EDGE_CURVE('',#6122,#6106,#3343,.T.);
#7726=EDGE_CURVE('',#6130,#6098,#3344,.T.);
#7727=EDGE_CURVE('',#6131,#6097,#3345,.T.);
#9782=ORIENTED_EDGE('',*,*,#7554,.T.);
#9783=ORIENTED_EDGE('',*,*,#7555,.T.);
#9784=ORIENTED_EDGE('',*,*,#7556,.T.);
#9785=ORIENTED_EDGE('',*,*,#7555,.F.);
#9786=ORIENTED_EDGE('',*,*,#7557,.F.);
#9787=ORIENTED_EDGE('',*,*,#7558,.F.);
#9788=ORIENTED_EDGE('',*,*,#7559,.F.);
#9789=ORIENTED_EDGE('',*,*,#7560,.F.);
#9790=ORIENTED_EDGE('',*,*,#7561,.F.);
#9791=ORIENTED_EDGE('',*,*,#7562,.F.);
#9792=ORIENTED_EDGE('',*,*,#7563,.F.);
#9793=ORIENTED_EDGE('',*,*,#7556,.F.);
#9794=ORIENTED_EDGE('',*,*,#7554,.F.);
#9795=ORIENTED_EDGE('',*,*,#7564,.T.);
#9796=ORIENTED_EDGE('',*,*,#7565,.F.);
#9797=ORIENTED_EDGE('',*,*,#7564,.F.);
#9798=ORIENTED_EDGE('',*,*,#7566,.T.);
#9799=ORIENTED_EDGE('',*,*,#7567,.T.);
#9800=ORIENTED_EDGE('',*,*,#7561,.T.);
#9801=ORIENTED_EDGE('',*,*,#7567,.F.);
#9802=ORIENTED_EDGE('',*,*,#7566,.F.);
#9803=ORIENTED_EDGE('',*,*,#7568,.T.);
#9804=ORIENTED_EDGE('',*,*,#7569,.F.);
#9805=ORIENTED_EDGE('',*,*,#7568,.F.);
#9806=ORIENTED_EDGE('',*,*,#7570,.T.);
#9807=ORIENTED_EDGE('',*,*,#7571,.T.);
#9808=ORIENTED_EDGE('',*,*,#7563,.T.);
#9809=ORIENTED_EDGE('',*,*,#7571,.F.);
#9810=ORIENTED_EDGE('',*,*,#7570,.F.);
#9811=ORIENTED_EDGE('',*,*,#7572,.T.);
#9812=ORIENTED_EDGE('',*,*,#7573,.F.);
#9813=ORIENTED_EDGE('',*,*,#7572,.F.);
#9814=ORIENTED_EDGE('',*,*,#7574,.T.);
#9815=ORIENTED_EDGE('',*,*,#7575,.T.);
#9816=ORIENTED_EDGE('',*,*,#7562,.T.);
#9817=ORIENTED_EDGE('',*,*,#7575,.F.);
#9818=ORIENTED_EDGE('',*,*,#7574,.F.);
#9819=ORIENTED_EDGE('',*,*,#7576,.T.);
#9820=ORIENTED_EDGE('',*,*,#7577,.F.);
#9821=ORIENTED_EDGE('',*,*,#7576,.F.);
#9822=ORIENTED_EDGE('',*,*,#7578,.T.);
#9823=ORIENTED_EDGE('',*,*,#7579,.T.);
#9824=ORIENTED_EDGE('',*,*,#7580,.T.);
#9825=ORIENTED_EDGE('',*,*,#7579,.F.);
#9826=ORIENTED_EDGE('',*,*,#7581,.F.);
#9827=ORIENTED_EDGE('',*,*,#7582,.F.);
#9828=ORIENTED_EDGE('',*,*,#7583,.T.);
#9829=ORIENTED_EDGE('',*,*,#7584,.F.);
#9830=ORIENTED_EDGE('',*,*,#7585,.F.);
#9831=ORIENTED_EDGE('',*,*,#7586,.F.);
#9832=ORIENTED_EDGE('',*,*,#7587,.F.);
#9833=ORIENTED_EDGE('',*,*,#7580,.F.);
#9834=ORIENTED_EDGE('',*,*,#7578,.F.);
#9835=ORIENTED_EDGE('',*,*,#7588,.T.);
#9836=ORIENTED_EDGE('',*,*,#7589,.F.);
#9837=ORIENTED_EDGE('',*,*,#7588,.F.);
#9838=ORIENTED_EDGE('',*,*,#7590,.T.);
#9839=ORIENTED_EDGE('',*,*,#7591,.T.);
#9840=ORIENTED_EDGE('',*,*,#7585,.T.);
#9841=ORIENTED_EDGE('',*,*,#7591,.F.);
#9842=ORIENTED_EDGE('',*,*,#7590,.F.);
#9843=ORIENTED_EDGE('',*,*,#7592,.T.);
#9844=ORIENTED_EDGE('',*,*,#7593,.F.);
#9845=ORIENTED_EDGE('',*,*,#7592,.F.);
#9846=ORIENTED_EDGE('',*,*,#7594,.T.);
#9847=ORIENTED_EDGE('',*,*,#7595,.T.);
#9848=ORIENTED_EDGE('',*,*,#7587,.T.);
#9849=ORIENTED_EDGE('',*,*,#7595,.F.);
#9850=ORIENTED_EDGE('',*,*,#7594,.F.);
#9851=ORIENTED_EDGE('',*,*,#7596,.T.);
#9852=ORIENTED_EDGE('',*,*,#7597,.F.);
#9853=ORIENTED_EDGE('',*,*,#7596,.F.);
#9854=ORIENTED_EDGE('',*,*,#7598,.T.);
#9855=ORIENTED_EDGE('',*,*,#7599,.T.);
#9856=ORIENTED_EDGE('',*,*,#7586,.T.);
#9857=ORIENTED_EDGE('',*,*,#7599,.F.);
#9858=ORIENTED_EDGE('',*,*,#7598,.F.);
#9859=ORIENTED_EDGE('',*,*,#7600,.T.);
#9860=ORIENTED_EDGE('',*,*,#7601,.F.);
#9861=ORIENTED_EDGE('',*,*,#7600,.F.);
#9862=ORIENTED_EDGE('',*,*,#7602,.T.);
#9863=ORIENTED_EDGE('',*,*,#7603,.T.);
#9864=ORIENTED_EDGE('',*,*,#7604,.T.);
#9865=ORIENTED_EDGE('',*,*,#7603,.F.);
#9866=ORIENTED_EDGE('',*,*,#7605,.F.);
#9867=ORIENTED_EDGE('',*,*,#7606,.F.);
#9868=ORIENTED_EDGE('',*,*,#7607,.F.);
#9869=ORIENTED_EDGE('',*,*,#7608,.F.);
#9870=ORIENTED_EDGE('',*,*,#7609,.F.);
#9871=ORIENTED_EDGE('',*,*,#7610,.F.);
#9872=ORIENTED_EDGE('',*,*,#7611,.F.);
#9873=ORIENTED_EDGE('',*,*,#7612,.F.);
#9874=ORIENTED_EDGE('',*,*,#7613,.F.);
#9875=ORIENTED_EDGE('',*,*,#7614,.F.);
#9876=ORIENTED_EDGE('',*,*,#7615,.F.);
#9877=ORIENTED_EDGE('',*,*,#7604,.F.);
#9878=ORIENTED_EDGE('',*,*,#7602,.F.);
#9879=ORIENTED_EDGE('',*,*,#7616,.T.);
#9880=ORIENTED_EDGE('',*,*,#7617,.T.);
#9881=ORIENTED_EDGE('',*,*,#7616,.F.);
#9882=ORIENTED_EDGE('',*,*,#7618,.T.);
#9883=ORIENTED_EDGE('',*,*,#7619,.T.);
#9884=ORIENTED_EDGE('',*,*,#7609,.T.);
#9885=ORIENTED_EDGE('',*,*,#7619,.F.);
#9886=ORIENTED_EDGE('',*,*,#7618,.F.);
#9887=ORIENTED_EDGE('',*,*,#7620,.T.);
#9888=ORIENTED_EDGE('',*,*,#7621,.T.);
#9889=ORIENTED_EDGE('',*,*,#7620,.F.);
#9890=ORIENTED_EDGE('',*,*,#7622,.T.);
#9891=ORIENTED_EDGE('',*,*,#7623,.T.);
#9892=ORIENTED_EDGE('',*,*,#7615,.T.);
#9893=ORIENTED_EDGE('',*,*,#7623,.F.);
#9894=ORIENTED_EDGE('',*,*,#7622,.F.);
#9895=ORIENTED_EDGE('',*,*,#7624,.T.);
#9896=ORIENTED_EDGE('',*,*,#7625,.T.);
#9897=ORIENTED_EDGE('',*,*,#7624,.F.);
#9898=ORIENTED_EDGE('',*,*,#7626,.T.);
#9899=ORIENTED_EDGE('',*,*,#7627,.T.);
#9900=ORIENTED_EDGE('',*,*,#7610,.T.);
#9901=ORIENTED_EDGE('',*,*,#7627,.F.);
#9902=ORIENTED_EDGE('',*,*,#7626,.F.);
#9903=ORIENTED_EDGE('',*,*,#7628,.T.);
#9904=ORIENTED_EDGE('',*,*,#7629,.T.);
#9905=ORIENTED_EDGE('',*,*,#7628,.F.);
#9906=ORIENTED_EDGE('',*,*,#7630,.T.);
#9907=ORIENTED_EDGE('',*,*,#7631,.T.);
#9908=ORIENTED_EDGE('',*,*,#7614,.T.);
#9909=ORIENTED_EDGE('',*,*,#7631,.F.);
#9910=ORIENTED_EDGE('',*,*,#7630,.F.);
#9911=ORIENTED_EDGE('',*,*,#7632,.T.);
#9912=ORIENTED_EDGE('',*,*,#7633,.T.);
#9913=ORIENTED_EDGE('',*,*,#7632,.F.);
#9914=ORIENTED_EDGE('',*,*,#7634,.T.);
#9915=ORIENTED_EDGE('',*,*,#7635,.T.);
#9916=ORIENTED_EDGE('',*,*,#7611,.T.);
#9917=ORIENTED_EDGE('',*,*,#7635,.F.);
#9918=ORIENTED_EDGE('',*,*,#7634,.F.);
#9919=ORIENTED_EDGE('',*,*,#7636,.T.);
#9920=ORIENTED_EDGE('',*,*,#7637,.T.);
#9921=ORIENTED_EDGE('',*,*,#7636,.F.);
#9922=ORIENTED_EDGE('',*,*,#7638,.T.);
#9923=ORIENTED_EDGE('',*,*,#7639,.T.);
#9924=ORIENTED_EDGE('',*,*,#7613,.T.);
#9925=ORIENTED_EDGE('',*,*,#7639,.F.);
#9926=ORIENTED_EDGE('',*,*,#7638,.F.);
#9927=ORIENTED_EDGE('',*,*,#7640,.T.);
#9928=ORIENTED_EDGE('',*,*,#7641,.T.);
#9929=ORIENTED_EDGE('',*,*,#7640,.F.);
#9930=ORIENTED_EDGE('',*,*,#7642,.T.);
#9931=ORIENTED_EDGE('',*,*,#7643,.T.);
#9932=ORIENTED_EDGE('',*,*,#7612,.T.);
#9933=ORIENTED_EDGE('',*,*,#7643,.F.);
#9934=ORIENTED_EDGE('',*,*,#7642,.F.);
#9935=ORIENTED_EDGE('',*,*,#7644,.T.);
#9936=ORIENTED_EDGE('',*,*,#7645,.T.);
#9937=ORIENTED_EDGE('',*,*,#7644,.F.);
#9938=ORIENTED_EDGE('',*,*,#7646,.T.);
#9939=ORIENTED_EDGE('',*,*,#7617,.F.);
#9940=ORIENTED_EDGE('',*,*,#7646,.F.);
#9941=ORIENTED_EDGE('',*,*,#7647,.T.);
#9942=ORIENTED_EDGE('',*,*,#7645,.F.);
#9943=ORIENTED_EDGE('',*,*,#7647,.F.);
#9944=ORIENTED_EDGE('',*,*,#7648,.T.);
#9945=ORIENTED_EDGE('',*,*,#7621,.F.);
#9946=ORIENTED_EDGE('',*,*,#7648,.F.);
#9947=ORIENTED_EDGE('',*,*,#7649,.T.);
#9948=ORIENTED_EDGE('',*,*,#7641,.F.);
#9949=ORIENTED_EDGE('',*,*,#7649,.F.);
#9950=ORIENTED_EDGE('',*,*,#7650,.T.);
#9951=ORIENTED_EDGE('',*,*,#7637,.F.);
#9952=ORIENTED_EDGE('',*,*,#7650,.F.);
#9953=ORIENTED_EDGE('',*,*,#7651,.T.);
#9954=ORIENTED_EDGE('',*,*,#7629,.F.);
#9955=ORIENTED_EDGE('',*,*,#7651,.F.);
#9956=ORIENTED_EDGE('',*,*,#7652,.T.);
#9957=ORIENTED_EDGE('',*,*,#7633,.F.);
#9958=ORIENTED_EDGE('',*,*,#7652,.F.);
#9959=ORIENTED_EDGE('',*,*,#7653,.T.);
#9960=ORIENTED_EDGE('',*,*,#7625,.F.);
#9961=ORIENTED_EDGE('',*,*,#7653,.F.);
#9962=ORIENTED_EDGE('',*,*,#7654,.T.);
#9963=ORIENTED_EDGE('',*,*,#7655,.T.);
#9964=ORIENTED_EDGE('',*,*,#7656,.T.);
#9965=ORIENTED_EDGE('',*,*,#7657,.T.);
#9966=ORIENTED_EDGE('',*,*,#7658,.T.);
#9967=ORIENTED_EDGE('',*,*,#7656,.F.);
#9968=ORIENTED_EDGE('',*,*,#7659,.T.);
#9969=ORIENTED_EDGE('',*,*,#7660,.T.);
#9970=ORIENTED_EDGE('',*,*,#7661,.T.);
#9971=ORIENTED_EDGE('',*,*,#7605,.T.);
#9972=ORIENTED_EDGE('',*,*,#7662,.T.);
#9973=ORIENTED_EDGE('',*,*,#7655,.F.);
#9974=ORIENTED_EDGE('',*,*,#7663,.T.);
#9975=ORIENTED_EDGE('',*,*,#7664,.T.);
#9976=ORIENTED_EDGE('',*,*,#7665,.T.);
#9977=ORIENTED_EDGE('',*,*,#7666,.T.);
#9978=ORIENTED_EDGE('',*,*,#7667,.F.);
#9979=ORIENTED_EDGE('',*,*,#7668,.T.);
#9980=ORIENTED_EDGE('',*,*,#7669,.F.);
#9981=ORIENTED_EDGE('',*,*,#7584,.T.);
#9982=ORIENTED_EDGE('',*,*,#7670,.T.);
#9983=ORIENTED_EDGE('',*,*,#7558,.T.);
#9984=ORIENTED_EDGE('',*,*,#7671,.F.);
#9985=ORIENTED_EDGE('',*,*,#7672,.T.);
#9986=ORIENTED_EDGE('',*,*,#7673,.F.);
#9987=ORIENTED_EDGE('',*,*,#7674,.T.);
#9988=ORIENTED_EDGE('',*,*,#7675,.T.);
#9989=ORIENTED_EDGE('',*,*,#7676,.T.);
#9990=ORIENTED_EDGE('',*,*,#7677,.T.);
#9991=ORIENTED_EDGE('',*,*,#7678,.F.);
#9992=ORIENTED_EDGE('',*,*,#7659,.F.);
#9993=ORIENTED_EDGE('',*,*,#7654,.F.);
#9994=ORIENTED_EDGE('',*,*,#7679,.T.);
#9995=ORIENTED_EDGE('',*,*,#7680,.F.);
#9996=ORIENTED_EDGE('',*,*,#7681,.T.);
#9997=ORIENTED_EDGE('',*,*,#7661,.F.);
#9998=ORIENTED_EDGE('',*,*,#7682,.F.);
#9999=ORIENTED_EDGE('',*,*,#7683,.T.);
#10000=ORIENTED_EDGE('',*,*,#7684,.F.);
#10001=ORIENTED_EDGE('',*,*,#7685,.F.);
#10002=ORIENTED_EDGE('',*,*,#7606,.T.);
#10003=ORIENTED_EDGE('',*,*,#7660,.F.);
#10004=ORIENTED_EDGE('',*,*,#7678,.T.);
#10005=ORIENTED_EDGE('',*,*,#7686,.T.);
#10006=ORIENTED_EDGE('',*,*,#7687,.T.);
#10007=ORIENTED_EDGE('',*,*,#7682,.T.);
#10008=ORIENTED_EDGE('',*,*,#7687,.F.);
#10009=ORIENTED_EDGE('',*,*,#7688,.F.);
#10010=ORIENTED_EDGE('',*,*,#7689,.F.);
#10011=ORIENTED_EDGE('',*,*,#7683,.F.);
#10012=ORIENTED_EDGE('',*,*,#7690,.T.);
#10013=ORIENTED_EDGE('',*,*,#7691,.T.);
#10014=ORIENTED_EDGE('',*,*,#7692,.T.);
#10015=ORIENTED_EDGE('',*,*,#7684,.T.);
#10016=ORIENTED_EDGE('',*,*,#7689,.T.);
#10017=ORIENTED_EDGE('',*,*,#7692,.F.);
#10018=ORIENTED_EDGE('',*,*,#7693,.T.);
#10019=ORIENTED_EDGE('',*,*,#7694,.T.);
#10020=ORIENTED_EDGE('',*,*,#7695,.T.);
#10021=ORIENTED_EDGE('',*,*,#7607,.T.);
#10022=ORIENTED_EDGE('',*,*,#7685,.T.);
#10023=ORIENTED_EDGE('',*,*,#7657,.F.);
#10024=ORIENTED_EDGE('',*,*,#7662,.F.);
#10025=ORIENTED_EDGE('',*,*,#7608,.T.);
#10026=ORIENTED_EDGE('',*,*,#7695,.F.);
#10027=ORIENTED_EDGE('',*,*,#7696,.F.);
#10028=ORIENTED_EDGE('',*,*,#7697,.T.);
#10029=ORIENTED_EDGE('',*,*,#7694,.F.);
#10030=ORIENTED_EDGE('',*,*,#7698,.T.);
#10031=ORIENTED_EDGE('',*,*,#7680,.T.);
#10032=ORIENTED_EDGE('',*,*,#7699,.T.);
#10033=ORIENTED_EDGE('',*,*,#7696,.T.);
#10034=ORIENTED_EDGE('',*,*,#7691,.F.);
#10035=ORIENTED_EDGE('',*,*,#7700,.T.);
#10036=ORIENTED_EDGE('',*,*,#7701,.T.);
#10037=ORIENTED_EDGE('',*,*,#7702,.T.);
#10038=ORIENTED_EDGE('',*,*,#7703,.T.);
#10039=ORIENTED_EDGE('',*,*,#7704,.F.);
#10040=ORIENTED_EDGE('',*,*,#7705,.T.);
#10041=ORIENTED_EDGE('',*,*,#7706,.F.);
#10042=ORIENTED_EDGE('',*,*,#7560,.T.);
#10043=ORIENTED_EDGE('',*,*,#7707,.T.);
#10044=ORIENTED_EDGE('',*,*,#7582,.T.);
#10045=ORIENTED_EDGE('',*,*,#7708,.F.);
#10046=ORIENTED_EDGE('',*,*,#7709,.T.);
#10047=ORIENTED_EDGE('',*,*,#7710,.F.);
#10048=ORIENTED_EDGE('',*,*,#7711,.T.);
#10049=ORIENTED_EDGE('',*,*,#7712,.T.);
#10050=ORIENTED_EDGE('',*,*,#7713,.T.);
#10051=ORIENTED_EDGE('',*,*,#7714,.T.);
#10052=ORIENTED_EDGE('',*,*,#7698,.F.);
#10053=ORIENTED_EDGE('',*,*,#7693,.F.);
#10054=ORIENTED_EDGE('',*,*,#7667,.T.);
#10055=ORIENTED_EDGE('',*,*,#7715,.T.);
#10056=ORIENTED_EDGE('',*,*,#7710,.T.);
#10057=ORIENTED_EDGE('',*,*,#7716,.T.);
#10058=ORIENTED_EDGE('',*,*,#7716,.F.);
#10059=ORIENTED_EDGE('',*,*,#7709,.F.);
#10060=ORIENTED_EDGE('',*,*,#7717,.F.);
#10061=ORIENTED_EDGE('',*,*,#7668,.F.);
#10062=ORIENTED_EDGE('',*,*,#7669,.T.);
#10063=ORIENTED_EDGE('',*,*,#7717,.T.);
#10064=ORIENTED_EDGE('',*,*,#7708,.T.);
#10065=ORIENTED_EDGE('',*,*,#7581,.T.);
#10066=ORIENTED_EDGE('',*,*,#7671,.T.);
#10067=ORIENTED_EDGE('',*,*,#7557,.T.);
#10068=ORIENTED_EDGE('',*,*,#7706,.T.);
#10069=ORIENTED_EDGE('',*,*,#7718,.T.);
#10070=ORIENTED_EDGE('',*,*,#7718,.F.);
#10071=ORIENTED_EDGE('',*,*,#7705,.F.);
#10072=ORIENTED_EDGE('',*,*,#7719,.F.);
#10073=ORIENTED_EDGE('',*,*,#7672,.F.);
#10074=ORIENTED_EDGE('',*,*,#7673,.T.);
#10075=ORIENTED_EDGE('',*,*,#7719,.T.);
#10076=ORIENTED_EDGE('',*,*,#7704,.T.);
#10077=ORIENTED_EDGE('',*,*,#7720,.T.);
#10078=ORIENTED_EDGE('',*,*,#7720,.F.);
#10079=ORIENTED_EDGE('',*,*,#7703,.F.);
#10080=ORIENTED_EDGE('',*,*,#7721,.T.);
#10081=ORIENTED_EDGE('',*,*,#7674,.F.);
#10082=ORIENTED_EDGE('',*,*,#7577,.T.);
#10083=ORIENTED_EDGE('',*,*,#7573,.T.);
#10084=ORIENTED_EDGE('',*,*,#7569,.T.);
#10085=ORIENTED_EDGE('',*,*,#7565,.T.);
#10086=ORIENTED_EDGE('',*,*,#7686,.F.);
#10087=ORIENTED_EDGE('',*,*,#7722,.T.);
#10088=ORIENTED_EDGE('',*,*,#7690,.F.);
#10089=ORIENTED_EDGE('',*,*,#7688,.T.);
#10090=ORIENTED_EDGE('',*,*,#7681,.F.);
#10091=ORIENTED_EDGE('',*,*,#7714,.F.);
#10092=ORIENTED_EDGE('',*,*,#7723,.T.);
#10093=ORIENTED_EDGE('',*,*,#7663,.F.);
#10094=ORIENTED_EDGE('',*,*,#7658,.F.);
#10095=ORIENTED_EDGE('',*,*,#7697,.F.);
#10096=ORIENTED_EDGE('',*,*,#7699,.F.);
#10097=ORIENTED_EDGE('',*,*,#7679,.F.);
#10098=ORIENTED_EDGE('',*,*,#7722,.F.);
#10099=ORIENTED_EDGE('',*,*,#7677,.F.);
#10100=ORIENTED_EDGE('',*,*,#7724,.F.);
#10101=ORIENTED_EDGE('',*,*,#7700,.F.);
#10102=ORIENTED_EDGE('',*,*,#7701,.F.);
#10103=ORIENTED_EDGE('',*,*,#7724,.T.);
#10104=ORIENTED_EDGE('',*,*,#7676,.F.);
#10105=ORIENTED_EDGE('',*,*,#7725,.F.);
#10106=ORIENTED_EDGE('',*,*,#7702,.F.);
#10107=ORIENTED_EDGE('',*,*,#7725,.T.);
#10108=ORIENTED_EDGE('',*,*,#7675,.F.);
#10109=ORIENTED_EDGE('',*,*,#7721,.F.);
#10110=ORIENTED_EDGE('',*,*,#7707,.F.);
#10111=ORIENTED_EDGE('',*,*,#7559,.T.);
#10112=ORIENTED_EDGE('',*,*,#7670,.F.);
#10113=ORIENTED_EDGE('',*,*,#7583,.F.);
#10114=ORIENTED_EDGE('',*,*,#7715,.F.);
#10115=ORIENTED_EDGE('',*,*,#7666,.F.);
#10116=ORIENTED_EDGE('',*,*,#7726,.F.);
#10117=ORIENTED_EDGE('',*,*,#7711,.F.);
#10118=ORIENTED_EDGE('',*,*,#7601,.T.);
#10119=ORIENTED_EDGE('',*,*,#7597,.T.);
#10120=ORIENTED_EDGE('',*,*,#7593,.T.);
#10121=ORIENTED_EDGE('',*,*,#7589,.T.);
#10122=ORIENTED_EDGE('',*,*,#7712,.F.);
#10123=ORIENTED_EDGE('',*,*,#7726,.T.);
#10124=ORIENTED_EDGE('',*,*,#7665,.F.);
#10125=ORIENTED_EDGE('',*,*,#7727,.F.);
#10126=ORIENTED_EDGE('',*,*,#7713,.F.);
#10127=ORIENTED_EDGE('',*,*,#7727,.T.);
#10128=ORIENTED_EDGE('',*,*,#7664,.F.);
#10129=ORIENTED_EDGE('',*,*,#7723,.F.);
#14238=CONICAL_SURFACE('',#15207,2.89999999999999,0.785398163397463);
#14239=CONICAL_SURFACE('',#15216,2.9,0.785398163397441);
#14240=CONICAL_SURFACE('',#15220,2.9,0.785398163397434);
#14241=CONICAL_SURFACE('',#15224,2.9,0.785398163397434);
#14242=CONICAL_SURFACE('',#15228,2.89999999999999,0.785398163397463);
#14243=CONICAL_SURFACE('',#15237,2.9,0.785398163397441);
#14244=CONICAL_SURFACE('',#15241,2.9,0.785398163397434);
#14245=CONICAL_SURFACE('',#15245,2.9,0.785398163397434);
#14246=CONICAL_SURFACE('',#15249,3.24999999999999,0.785398163397438);
#14247=CONICAL_SURFACE('',#15262,3.24999999999999,0.785398163397438);
#14248=CONICAL_SURFACE('',#15266,3.25,0.785398163397449);
#14249=CONICAL_SURFACE('',#15270,3.25,0.785398163397449);
#14250=CONICAL_SURFACE('',#15274,3.25,0.785398163397449);
#14251=CONICAL_SURFACE('',#15278,3.25,0.785398163397449);
#14252=CONICAL_SURFACE('',#15282,3.24999999999999,0.785398163397438);
#14253=CONICAL_SURFACE('',#15286,3.24999999999999,0.785398163397438);
#14254=CONICAL_SURFACE('',#15290,1.525,1.02974425867665);
#14255=CONICAL_SURFACE('',#15291,1.525,1.02974425867665);
#14256=CONICAL_SURFACE('',#15292,1.525,1.02974425867666);
#14257=CONICAL_SURFACE('',#15293,1.525,1.02974425867666);
#14258=CONICAL_SURFACE('',#15294,1.525,1.02974425867665);
#14259=CONICAL_SURFACE('',#15295,1.525,1.02974425867665);
#14260=CONICAL_SURFACE('',#15296,1.525,1.02974425867665);
#14261=CONICAL_SURFACE('',#15297,1.525,1.02974425867665);
#14341=ADVANCED_FACE('',(#1606),#14238,.F.);
#14342=ADVANCED_FACE('',(#1607,#1083,#1084,#1085,#1086),#1211,.T.);
#14343=ADVANCED_FACE('',(#1608),#851,.F.);
#14344=ADVANCED_FACE('',(#1609),#14239,.F.);
#14345=ADVANCED_FACE('',(#1610),#852,.F.);
#14346=ADVANCED_FACE('',(#1611),#14240,.F.);
#14347=ADVANCED_FACE('',(#1612),#853,.F.);
#14348=ADVANCED_FACE('',(#1613),#14241,.F.);
#14349=ADVANCED_FACE('',(#1614),#854,.F.);
#14350=ADVANCED_FACE('',(#1615),#14242,.F.);
#14351=ADVANCED_FACE('',(#1616,#1087,#1088,#1089,#1090),#1212,.T.);
#14352=ADVANCED_FACE('',(#1617),#855,.F.);
#14353=ADVANCED_FACE('',(#1618),#14243,.F.);
#14354=ADVANCED_FACE('',(#1619),#856,.F.);
#14355=ADVANCED_FACE('',(#1620),#14244,.F.);
#14356=ADVANCED_FACE('',(#1621),#857,.F.);
#14357=ADVANCED_FACE('',(#1622),#14245,.F.);
#14358=ADVANCED_FACE('',(#1623),#858,.F.);
#14359=ADVANCED_FACE('',(#1624),#14246,.F.);
#14360=ADVANCED_FACE('',(#1625,#1091,#1092,#1093,#1094,#1095,#1096,#1097,
#1098),#1213,.T.);
#14361=ADVANCED_FACE('',(#1626),#859,.F.);
#14362=ADVANCED_FACE('',(#1627),#14247,.F.);
#14363=ADVANCED_FACE('',(#1628),#860,.F.);
#14364=ADVANCED_FACE('',(#1629),#14248,.F.);
#14365=ADVANCED_FACE('',(#1630),#861,.F.);
#14366=ADVANCED_FACE('',(#1631),#14249,.F.);
#14367=ADVANCED_FACE('',(#1632),#862,.F.);
#14368=ADVANCED_FACE('',(#1633),#14250,.F.);
#14369=ADVANCED_FACE('',(#1634),#863,.F.);
#14370=ADVANCED_FACE('',(#1635),#14251,.F.);
#14371=ADVANCED_FACE('',(#1636),#864,.F.);
#14372=ADVANCED_FACE('',(#1637),#14252,.F.);
#14373=ADVANCED_FACE('',(#1638),#865,.F.);
#14374=ADVANCED_FACE('',(#1639),#14253,.F.);
#14375=ADVANCED_FACE('',(#1640),#866,.F.);
#14376=ADVANCED_FACE('',(#1641),#14254,.F.);
#14377=ADVANCED_FACE('',(#1642),#14255,.F.);
#14378=ADVANCED_FACE('',(#1643),#14256,.F.);
#14379=ADVANCED_FACE('',(#1644),#14257,.F.);
#14380=ADVANCED_FACE('',(#1645),#14258,.F.);
#14381=ADVANCED_FACE('',(#1646),#14259,.F.);
#14382=ADVANCED_FACE('',(#1647),#14260,.F.);
#14383=ADVANCED_FACE('',(#1648),#14261,.F.);
#14384=ADVANCED_FACE('',(#1649),#1214,.T.);
#14385=ADVANCED_FACE('',(#1650),#1215,.T.);
#14386=ADVANCED_FACE('',(#1651),#1216,.T.);
#14387=ADVANCED_FACE('',(#1652),#1217,.T.);
#14388=ADVANCED_FACE('',(#1653),#1218,.T.);
#14389=ADVANCED_FACE('',(#1654),#1219,.T.);
#14390=ADVANCED_FACE('',(#1655),#1220,.T.);
#14391=ADVANCED_FACE('',(#1656),#1221,.T.);
#14392=ADVANCED_FACE('',(#1657),#1222,.T.);
#14393=ADVANCED_FACE('',(#1658),#1223,.T.);
#14394=ADVANCED_FACE('',(#1659),#1224,.T.);
#14395=ADVANCED_FACE('',(#1660),#1225,.F.);
#14396=ADVANCED_FACE('',(#1661),#1226,.T.);
#14397=ADVANCED_FACE('',(#1662),#1227,.T.);
#14398=ADVANCED_FACE('',(#1663),#1228,.T.);
#14399=ADVANCED_FACE('',(#1664),#1229,.T.);
#14400=ADVANCED_FACE('',(#1665),#1230,.T.);
#14401=ADVANCED_FACE('',(#1666),#1231,.T.);
#14402=ADVANCED_FACE('',(#1667,#1099,#1100,#1101,#1102),#1232,.T.);
#14403=ADVANCED_FACE('',(#1668),#1233,.T.);
#14404=ADVANCED_FACE('',(#1669),#1234,.T.);
#14405=ADVANCED_FACE('',(#1670),#1235,.T.);
#14406=ADVANCED_FACE('',(#1671),#1236,.T.);
#14407=ADVANCED_FACE('',(#1672),#1237,.T.);
#14408=ADVANCED_FACE('',(#1673),#1238,.T.);
#14409=ADVANCED_FACE('',(#1674),#1239,.T.);
#14410=ADVANCED_FACE('',(#1675,#1103,#1104,#1105,#1106),#1240,.T.);
#14411=ADVANCED_FACE('',(#1676),#1241,.T.);
#14412=ADVANCED_FACE('',(#1677),#1242,.T.);
#15084=CLOSED_SHELL('',(#14341,#14342,#14343,#14344,#14345,#14346,#14347,
#14348,#14349,#14350,#14351,#14352,#14353,#14354,#14355,#14356,#14357,#14358,
#14359,#14360,#14361,#14362,#14363,#14364,#14365,#14366,#14367,#14368,#14369,
#14370,#14371,#14372,#14373,#14374,#14375,#14376,#14377,#14378,#14379,#14380,
#14381,#14382,#14383,#14384,#14385,#14386,#14387,#14388,#14389,#14390,#14391,
#14392,#14393,#14394,#14395,#14396,#14397,#14398,#14399,#14400,#14401,#14402,
#14403,#14404,#14405,#14406,#14407,#14408,#14409,#14410,#14411,#14412));
#15206=AXIS2_PLACEMENT_3D('',#20563,#16622,#16623);
#15207=AXIS2_PLACEMENT_3D('',#20564,#16624,#16625);
#15208=AXIS2_PLACEMENT_3D('',#20566,#16626,#16627);
#15209=AXIS2_PLACEMENT_3D('',#20569,#16629,#16630);
#15210=AXIS2_PLACEMENT_3D('',#20570,#16631,#16632);
#15211=AXIS2_PLACEMENT_3D('',#20580,#16637,#16638);
#15212=AXIS2_PLACEMENT_3D('',#20582,#16639,#16640);
#15213=AXIS2_PLACEMENT_3D('',#20584,#16641,#16642);
#15214=AXIS2_PLACEMENT_3D('',#20585,#16643,#16644);
#15215=AXIS2_PLACEMENT_3D('',#20588,#16646,#16647);
#15216=AXIS2_PLACEMENT_3D('',#20589,#16648,#16649);
#15217=AXIS2_PLACEMENT_3D('',#20591,#16650,#16651);
#15218=AXIS2_PLACEMENT_3D('',#20593,#16653,#16654);
#15219=AXIS2_PLACEMENT_3D('',#20596,#16656,#16657);
#15220=AXIS2_PLACEMENT_3D('',#20597,#16658,#16659);
#15221=AXIS2_PLACEMENT_3D('',#20599,#16660,#16661);
#15222=AXIS2_PLACEMENT_3D('',#20601,#16663,#16664);
#15223=AXIS2_PLACEMENT_3D('',#20604,#16666,#16667);
#15224=AXIS2_PLACEMENT_3D('',#20605,#16668,#16669);
#15225=AXIS2_PLACEMENT_3D('',#20607,#16670,#16671);
#15226=AXIS2_PLACEMENT_3D('',#20609,#16673,#16674);
#15227=AXIS2_PLACEMENT_3D('',#20612,#16676,#16677);
#15228=AXIS2_PLACEMENT_3D('',#20613,#16678,#16679);
#15229=AXIS2_PLACEMENT_3D('',#20615,#16680,#16681);
#15230=AXIS2_PLACEMENT_3D('',#20618,#16683,#16684);
#15231=AXIS2_PLACEMENT_3D('',#20619,#16685,#16686);
#15232=AXIS2_PLACEMENT_3D('',#20629,#16691,#16692);
#15233=AXIS2_PLACEMENT_3D('',#20631,#16693,#16694);
#15234=AXIS2_PLACEMENT_3D('',#20633,#16695,#16696);
#15235=AXIS2_PLACEMENT_3D('',#20634,#16697,#16698);
#15236=AXIS2_PLACEMENT_3D('',#20637,#16700,#16701);
#15237=AXIS2_PLACEMENT_3D('',#20638,#16702,#16703);
#15238=AXIS2_PLACEMENT_3D('',#20640,#16704,#16705);
#15239=AXIS2_PLACEMENT_3D('',#20642,#16707,#16708);
#15240=AXIS2_PLACEMENT_3D('',#20645,#16710,#16711);
#15241=AXIS2_PLACEMENT_3D('',#20646,#16712,#16713);
#15242=AXIS2_PLACEMENT_3D('',#20648,#16714,#16715);
#15243=AXIS2_PLACEMENT_3D('',#20650,#16717,#16718);
#15244=AXIS2_PLACEMENT_3D('',#20653,#16720,#16721);
#15245=AXIS2_PLACEMENT_3D('',#20654,#16722,#16723);
#15246=AXIS2_PLACEMENT_3D('',#20656,#16724,#16725);
#15247=AXIS2_PLACEMENT_3D('',#20658,#16727,#16728);
#15248=AXIS2_PLACEMENT_3D('',#20661,#16730,#16731);
#15249=AXIS2_PLACEMENT_3D('',#20662,#16732,#16733);
#15250=AXIS2_PLACEMENT_3D('',#20664,#16734,#16735);
#15251=AXIS2_PLACEMENT_3D('',#20667,#16737,#16738);
#15252=AXIS2_PLACEMENT_3D('',#20668,#16739,#16740);
#15253=AXIS2_PLACEMENT_3D('',#20678,#16745,#16746);
#15254=AXIS2_PLACEMENT_3D('',#20680,#16747,#16748);
#15255=AXIS2_PLACEMENT_3D('',#20682,#16749,#16750);
#15256=AXIS2_PLACEMENT_3D('',#20684,#16751,#16752);
#15257=AXIS2_PLACEMENT_3D('',#20686,#16753,#16754);
#15258=AXIS2_PLACEMENT_3D('',#20688,#16755,#16756);
#15259=AXIS2_PLACEMENT_3D('',#20690,#16757,#16758);
#15260=AXIS2_PLACEMENT_3D('',#20691,#16759,#16760);
#15261=AXIS2_PLACEMENT_3D('',#20694,#16762,#16763);
#15262=AXIS2_PLACEMENT_3D('',#20695,#16764,#16765);
#15263=AXIS2_PLACEMENT_3D('',#20697,#16766,#16767);
#15264=AXIS2_PLACEMENT_3D('',#20699,#16769,#16770);
#15265=AXIS2_PLACEMENT_3D('',#20702,#16772,#16773);
#15266=AXIS2_PLACEMENT_3D('',#20703,#16774,#16775);
#15267=AXIS2_PLACEMENT_3D('',#20705,#16776,#16777);
#15268=AXIS2_PLACEMENT_3D('',#20707,#16779,#16780);
#15269=AXIS2_PLACEMENT_3D('',#20710,#16782,#16783);
#15270=AXIS2_PLACEMENT_3D('',#20711,#16784,#16785);
#15271=AXIS2_PLACEMENT_3D('',#20713,#16786,#16787);
#15272=AXIS2_PLACEMENT_3D('',#20715,#16789,#16790);
#15273=AXIS2_PLACEMENT_3D('',#20718,#16792,#16793);
#15274=AXIS2_PLACEMENT_3D('',#20719,#16794,#16795);
#15275=AXIS2_PLACEMENT_3D('',#20721,#16796,#16797);
#15276=AXIS2_PLACEMENT_3D('',#20723,#16799,#16800);
#15277=AXIS2_PLACEMENT_3D('',#20726,#16802,#16803);
#15278=AXIS2_PLACEMENT_3D('',#20727,#16804,#16805);
#15279=AXIS2_PLACEMENT_3D('',#20729,#16806,#16807);
#15280=AXIS2_PLACEMENT_3D('',#20731,#16809,#16810);
#15281=AXIS2_PLACEMENT_3D('',#20734,#16812,#16813);
#15282=AXIS2_PLACEMENT_3D('',#20735,#16814,#16815);
#15283=AXIS2_PLACEMENT_3D('',#20737,#16816,#16817);
#15284=AXIS2_PLACEMENT_3D('',#20739,#16819,#16820);
#15285=AXIS2_PLACEMENT_3D('',#20742,#16822,#16823);
#15286=AXIS2_PLACEMENT_3D('',#20743,#16824,#16825);
#15287=AXIS2_PLACEMENT_3D('',#20745,#16826,#16827);
#15288=AXIS2_PLACEMENT_3D('',#20747,#16829,#16830);
#15289=AXIS2_PLACEMENT_3D('',#20750,#16832,#16833);
#15290=AXIS2_PLACEMENT_3D('',#20751,#16834,#16835);
#15291=AXIS2_PLACEMENT_3D('',#20754,#16837,#16838);
#15292=AXIS2_PLACEMENT_3D('',#20757,#16840,#16841);
#15293=AXIS2_PLACEMENT_3D('',#20760,#16843,#16844);
#15294=AXIS2_PLACEMENT_3D('',#20763,#16846,#16847);
#15295=AXIS2_PLACEMENT_3D('',#20766,#16849,#16850);
#15296=AXIS2_PLACEMENT_3D('',#20769,#16852,#16853);
#15297=AXIS2_PLACEMENT_3D('',#20772,#16855,#16856);
#15298=AXIS2_PLACEMENT_3D('',#20775,#16858,#16859);
#15299=AXIS2_PLACEMENT_3D('',#20786,#16865,#16866);
#15300=AXIS2_PLACEMENT_3D('',#20793,#16871,#16872);
#15301=AXIS2_PLACEMENT_3D('',#20823,#16889,#16890);
#15302=AXIS2_PLACEMENT_3D('',#20829,#16894,#16895);
#15303=AXIS2_PLACEMENT_3D('',#20837,#16900,#16901);
#15304=AXIS2_PLACEMENT_3D('',#20841,#16904,#16905);
#15305=AXIS2_PLACEMENT_3D('',#20845,#16908,#16909);
#15306=AXIS2_PLACEMENT_3D('',#20851,#16913,#16914);
#15307=AXIS2_PLACEMENT_3D('',#20857,#16918,#16919);
#15308=AXIS2_PLACEMENT_3D('',#20861,#16922,#16923);
#15309=AXIS2_PLACEMENT_3D('',#20864,#16926,#16927);
#15310=AXIS2_PLACEMENT_3D('',#20892,#16943,#16944);
#15311=AXIS2_PLACEMENT_3D('',#20895,#16947,#16948);
#15312=AXIS2_PLACEMENT_3D('',#20897,#16950,#16951);
#15313=AXIS2_PLACEMENT_3D('',#20898,#16952,#16953);
#15314=AXIS2_PLACEMENT_3D('',#20900,#16955,#16956);
#15315=AXIS2_PLACEMENT_3D('',#20902,#16958,#16959);
#15316=AXIS2_PLACEMENT_3D('',#20904,#16961,#16962);
#15317=AXIS2_PLACEMENT_3D('',#20906,#16964,#16965);
#15318=AXIS2_PLACEMENT_3D('',#20908,#16967,#16968);
#15319=AXIS2_PLACEMENT_3D('',#20910,#16970,#16971);
#15320=AXIS2_PLACEMENT_3D('',#20911,#16972,#16973);
#15321=AXIS2_PLACEMENT_3D('',#20913,#16975,#16976);
#15322=AXIS2_PLACEMENT_3D('',#20915,#16978,#16979);
#15323=AXIS2_PLACEMENT_3D('',#20916,#16980,#16981);
#15324=AXIS2_PLACEMENT_3D('',#20917,#16982,#16983);
#15325=AXIS2_PLACEMENT_3D('',#20919,#16985,#16986);
#15326=AXIS2_PLACEMENT_3D('',#20921,#16988,#16989);
#16622=DIRECTION('axis',(0.,0.,1.));
#16623=DIRECTION('refdir',(1.,0.,0.));
#16624=DIRECTION('center_axis',(0.,0.,-1.));
#16625=DIRECTION('ref_axis',(1.,0.,0.));
#16626=DIRECTION('center_axis',(0.,0.,1.));
#16627=DIRECTION('ref_axis',(1.,0.,0.));
#16628=DIRECTION('',(-0.707106781186558,8.65956056235506E-17,-0.707106781186537));
#16629=DIRECTION('center_axis',(0.,0.,-1.));
#16630=DIRECTION('ref_axis',(1.,0.,0.));
#16631=DIRECTION('center_axis',(0.,0.,-1.));
#16632=DIRECTION('ref_axis',(0.,1.,0.));
#16633=DIRECTION('',(-1.,0.,0.));
#16634=DIRECTION('',(0.,1.,0.));
#16635=DIRECTION('',(1.,0.,0.));
#16636=DIRECTION('',(0.,-1.,0.));
#16637=DIRECTION('center_axis',(0.,0.,-1.));
#16638=DIRECTION('ref_axis',(1.,0.,0.));
#16639=DIRECTION('center_axis',(0.,0.,-1.));
#16640=DIRECTION('ref_axis',(1.,0.,0.));
#16641=DIRECTION('center_axis',(0.,0.,-1.));
#16642=DIRECTION('ref_axis',(1.,0.,0.));
#16643=DIRECTION('center_axis',(0.,0.,1.));
#16644=DIRECTION('ref_axis',(1.,0.,0.));
#16645=DIRECTION('',(0.,0.,1.));
#16646=DIRECTION('center_axis',(0.,0.,-1.));
#16647=DIRECTION('ref_axis',(1.,0.,0.));
#16648=DIRECTION('center_axis',(0.,0.,-1.));
#16649=DIRECTION('ref_axis',(1.,0.,0.));
#16650=DIRECTION('center_axis',(0.,0.,1.));
#16651=DIRECTION('ref_axis',(1.,0.,0.));
#16652=DIRECTION('',(-0.707106781186542,8.65956056235487E-17,-0.707106781186553));
#16653=DIRECTION('center_axis',(0.,0.,1.));
#16654=DIRECTION('ref_axis',(1.,0.,0.));
#16655=DIRECTION('',(0.,0.,1.));
#16656=DIRECTION('center_axis',(0.,0.,-1.));
#16657=DIRECTION('ref_axis',(1.,0.,0.));
#16658=DIRECTION('center_axis',(0.,0.,-1.));
#16659=DIRECTION('ref_axis',(1.,0.,0.));
#16660=DIRECTION('center_axis',(0.,0.,1.));
#16661=DIRECTION('ref_axis',(1.,0.,0.));
#16662=DIRECTION('',(-0.707106781186537,8.65956056235481E-17,-0.707106781186558));
#16663=DIRECTION('center_axis',(0.,0.,1.));
#16664=DIRECTION('ref_axis',(1.,0.,0.));
#16665=DIRECTION('',(0.,0.,1.));
#16666=DIRECTION('center_axis',(0.,0.,-1.));
#16667=DIRECTION('ref_axis',(1.,0.,0.));
#16668=DIRECTION('center_axis',(0.,0.,-1.));
#16669=DIRECTION('ref_axis',(1.,0.,0.));
#16670=DIRECTION('center_axis',(0.,0.,1.));
#16671=DIRECTION('ref_axis',(1.,0.,0.));
#16672=DIRECTION('',(-0.707106781186537,8.65956056235481E-17,-0.707106781186558));
#16673=DIRECTION('center_axis',(0.,0.,1.));
#16674=DIRECTION('ref_axis',(1.,0.,0.));
#16675=DIRECTION('',(0.,0.,1.));
#16676=DIRECTION('center_axis',(0.,0.,-1.));
#16677=DIRECTION('ref_axis',(1.,0.,0.));
#16678=DIRECTION('center_axis',(0.,0.,1.));
#16679=DIRECTION('ref_axis',(1.,0.,0.));
#16680=DIRECTION('center_axis',(0.,0.,-1.));
#16681=DIRECTION('ref_axis',(1.,0.,0.));
#16682=DIRECTION('',(-0.707106781186558,-8.65956056235506E-17,0.707106781186537));
#16683=DIRECTION('center_axis',(0.,0.,1.));
#16684=DIRECTION('ref_axis',(1.,0.,0.));
#16685=DIRECTION('center_axis',(0.,0.,1.));
#16686=DIRECTION('ref_axis',(0.,-1.,0.));
#16687=DIRECTION('',(1.,0.,0.));
#16688=DIRECTION('',(0.,1.,0.));
#16689=DIRECTION('',(1.,0.,0.));
#16690=DIRECTION('',(0.,-1.,0.));
#16691=DIRECTION('center_axis',(0.,0.,1.));
#16692=DIRECTION('ref_axis',(1.,0.,0.));
#16693=DIRECTION('center_axis',(0.,0.,1.));
#16694=DIRECTION('ref_axis',(1.,0.,0.));
#16695=DIRECTION('center_axis',(0.,0.,1.));
#16696=DIRECTION('ref_axis',(1.,0.,0.));
#16697=DIRECTION('center_axis',(0.,0.,-1.));
#16698=DIRECTION('ref_axis',(1.,0.,0.));
#16699=DIRECTION('',(0.,0.,-1.));
#16700=DIRECTION('center_axis',(0.,0.,1.));
#16701=DIRECTION('ref_axis',(1.,0.,0.));
#16702=DIRECTION('center_axis',(0.,0.,1.));
#16703=DIRECTION('ref_axis',(1.,0.,0.));
#16704=DIRECTION('center_axis',(0.,0.,-1.));
#16705=DIRECTION('ref_axis',(1.,0.,0.));
#16706=DIRECTION('',(-0.707106781186542,-8.65956056235487E-17,0.707106781186553));
#16707=DIRECTION('center_axis',(0.,0.,-1.));
#16708=DIRECTION('ref_axis',(1.,0.,0.));
#16709=DIRECTION('',(0.,0.,-1.));
#16710=DIRECTION('center_axis',(0.,0.,1.));
#16711=DIRECTION('ref_axis',(1.,0.,0.));
#16712=DIRECTION('center_axis',(0.,0.,1.));
#16713=DIRECTION('ref_axis',(1.,0.,0.));
#16714=DIRECTION('center_axis',(0.,0.,-1.));
#16715=DIRECTION('ref_axis',(1.,0.,0.));
#16716=DIRECTION('',(-0.707106781186537,-8.65956056235481E-17,0.707106781186558));
#16717=DIRECTION('center_axis',(0.,0.,-1.));
#16718=DIRECTION('ref_axis',(1.,0.,0.));
#16719=DIRECTION('',(0.,0.,-1.));
#16720=DIRECTION('center_axis',(0.,0.,1.));
#16721=DIRECTION('ref_axis',(1.,0.,0.));
#16722=DIRECTION('center_axis',(0.,0.,1.));
#16723=DIRECTION('ref_axis',(1.,0.,0.));
#16724=DIRECTION('center_axis',(0.,0.,-1.));
#16725=DIRECTION('ref_axis',(1.,0.,0.));
#16726=DIRECTION('',(-0.707106781186537,-8.65956056235481E-17,0.707106781186558));
#16727=DIRECTION('center_axis',(0.,0.,-1.));
#16728=DIRECTION('ref_axis',(1.,0.,0.));
#16729=DIRECTION('',(0.,0.,-1.));
#16730=DIRECTION('center_axis',(0.,0.,1.));
#16731=DIRECTION('ref_axis',(1.,0.,0.));
#16732=DIRECTION('center_axis',(0.,-1.,0.));
#16733=DIRECTION('ref_axis',(1.,0.,0.));
#16734=DIRECTION('center_axis',(0.,1.,0.));
#16735=DIRECTION('ref_axis',(1.,0.,0.));
#16736=DIRECTION('',(-0.70710678118654,-0.707106781186555,-8.65956056235484E-17));
#16737=DIRECTION('center_axis',(0.,-1.,0.));
#16738=DIRECTION('ref_axis',(1.,0.,0.));
#16739=DIRECTION('center_axis',(0.,-1.,0.));
#16740=DIRECTION('ref_axis',(0.,0.,-1.));
#16741=DIRECTION('',(0.,0.,-1.));
#16742=DIRECTION('',(1.,0.,0.));
#16743=DIRECTION('',(0.,0.,1.));
#16744=DIRECTION('',(-1.,0.,0.));
#16745=DIRECTION('center_axis',(0.,-1.,0.));
#16746=DIRECTION('ref_axis',(1.,0.,0.));
#16747=DIRECTION('center_axis',(0.,-1.,0.));
#16748=DIRECTION('ref_axis',(1.,0.,0.));
#16749=DIRECTION('center_axis',(0.,-1.,0.));
#16750=DIRECTION('ref_axis',(1.,0.,0.));
#16751=DIRECTION('center_axis',(0.,-1.,0.));
#16752=DIRECTION('ref_axis',(1.,0.,0.));
#16753=DIRECTION('center_axis',(0.,-1.,0.));
#16754=DIRECTION('ref_axis',(1.,0.,0.));
#16755=DIRECTION('center_axis',(0.,-1.,0.));
#16756=DIRECTION('ref_axis',(1.,0.,0.));
#16757=DIRECTION('center_axis',(0.,-1.,0.));
#16758=DIRECTION('ref_axis',(1.,0.,0.));
#16759=DIRECTION('center_axis',(0.,1.,0.));
#16760=DIRECTION('ref_axis',(1.,0.,0.));
#16761=DIRECTION('',(0.,1.,0.));
#16762=DIRECTION('center_axis',(0.,1.,0.));
#16763=DIRECTION('ref_axis',(1.,0.,0.));
#16764=DIRECTION('center_axis',(0.,-1.,0.));
#16765=DIRECTION('ref_axis',(1.,0.,0.));
#16766=DIRECTION('center_axis',(0.,1.,0.));
#16767=DIRECTION('ref_axis',(1.,0.,0.));
#16768=DIRECTION('',(-0.70710678118654,-0.707106781186555,-8.65956056235484E-17));
#16769=DIRECTION('center_axis',(0.,1.,0.));
#16770=DIRECTION('ref_axis',(1.,0.,0.));
#16771=DIRECTION('',(0.,1.,0.));
#16772=DIRECTION('center_axis',(0.,1.,0.));
#16773=DIRECTION('ref_axis',(1.,0.,0.));
#16774=DIRECTION('center_axis',(0.,-1.,0.));
#16775=DIRECTION('ref_axis',(1.,0.,0.));
#16776=DIRECTION('center_axis',(0.,1.,0.));
#16777=DIRECTION('ref_axis',(1.,0.,0.));
#16778=DIRECTION('',(-0.707106781186548,-0.707106781186547,-8.65956056235494E-17));
#16779=DIRECTION('center_axis',(0.,1.,0.));
#16780=DIRECTION('ref_axis',(1.,0.,0.));
#16781=DIRECTION('',(0.,1.,0.));
#16782=DIRECTION('center_axis',(0.,1.,0.));
#16783=DIRECTION('ref_axis',(1.,0.,0.));
#16784=DIRECTION('center_axis',(0.,-1.,0.));
#16785=DIRECTION('ref_axis',(1.,0.,0.));
#16786=DIRECTION('center_axis',(0.,1.,0.));
#16787=DIRECTION('ref_axis',(1.,0.,0.));
#16788=DIRECTION('',(-0.707106781186548,-0.707106781186547,-8.65956056235494E-17));
#16789=DIRECTION('center_axis',(0.,1.,0.));
#16790=DIRECTION('ref_axis',(1.,0.,0.));
#16791=DIRECTION('',(0.,1.,0.));
#16792=DIRECTION('center_axis',(0.,1.,0.));
#16793=DIRECTION('ref_axis',(1.,0.,0.));
#16794=DIRECTION('center_axis',(0.,-1.,0.));
#16795=DIRECTION('ref_axis',(1.,0.,0.));
#16796=DIRECTION('center_axis',(0.,1.,0.));
#16797=DIRECTION('ref_axis',(1.,0.,0.));
#16798=DIRECTION('',(-0.707106781186548,-0.707106781186547,-8.65956056235494E-17));
#16799=DIRECTION('center_axis',(0.,1.,0.));
#16800=DIRECTION('ref_axis',(1.,0.,0.));
#16801=DIRECTION('',(0.,1.,0.));
#16802=DIRECTION('center_axis',(0.,1.,0.));
#16803=DIRECTION('ref_axis',(1.,0.,0.));
#16804=DIRECTION('center_axis',(0.,-1.,0.));
#16805=DIRECTION('ref_axis',(1.,0.,0.));
#16806=DIRECTION('center_axis',(0.,1.,0.));
#16807=DIRECTION('ref_axis',(1.,0.,0.));
#16808=DIRECTION('',(-0.707106781186548,-0.707106781186547,-8.65956056235494E-17));
#16809=DIRECTION('center_axis',(0.,1.,0.));
#16810=DIRECTION('ref_axis',(1.,0.,0.));
#16811=DIRECTION('',(0.,1.,0.));
#16812=DIRECTION('center_axis',(0.,1.,0.));
#16813=DIRECTION('ref_axis',(1.,0.,0.));
#16814=DIRECTION('center_axis',(0.,-1.,0.));
#16815=DIRECTION('ref_axis',(1.,0.,0.));
#16816=DIRECTION('center_axis',(0.,1.,0.));
#16817=DIRECTION('ref_axis',(1.,0.,0.));
#16818=DIRECTION('',(-0.70710678118654,-0.707106781186555,-8.65956056235484E-17));
#16819=DIRECTION('center_axis',(0.,1.,0.));
#16820=DIRECTION('ref_axis',(1.,0.,0.));
#16821=DIRECTION('',(0.,1.,0.));
#16822=DIRECTION('center_axis',(0.,1.,0.));
#16823=DIRECTION('ref_axis',(1.,0.,0.));
#16824=DIRECTION('center_axis',(0.,-1.,0.));
#16825=DIRECTION('ref_axis',(1.,0.,0.));
#16826=DIRECTION('center_axis',(0.,1.,0.));
#16827=DIRECTION('ref_axis',(1.,0.,0.));
#16828=DIRECTION('',(-0.70710678118654,-0.707106781186555,-8.65956056235484E-17));
#16829=DIRECTION('center_axis',(0.,1.,0.));
#16830=DIRECTION('ref_axis',(1.,0.,0.));
#16831=DIRECTION('',(0.,1.,0.));
#16832=DIRECTION('center_axis',(0.,1.,0.));
#16833=DIRECTION('ref_axis',(1.,0.,0.));
#16834=DIRECTION('center_axis',(0.,-1.,0.));
#16835=DIRECTION('ref_axis',(1.,0.,0.));
#16836=DIRECTION('',(-0.85716730070211,-0.515038074910058,-1.04972719113862E-16));
#16837=DIRECTION('center_axis',(0.,-1.,0.));
#16838=DIRECTION('ref_axis',(1.,0.,0.));
#16839=DIRECTION('',(-0.85716730070211,-0.515038074910058,-1.04972719113862E-16));
#16840=DIRECTION('center_axis',(0.,-1.,0.));
#16841=DIRECTION('ref_axis',(1.,0.,0.));
#16842=DIRECTION('',(-0.857167300702115,-0.515038074910049,-1.04972719113862E-16));
#16843=DIRECTION('center_axis',(0.,-1.,0.));
#16844=DIRECTION('ref_axis',(1.,0.,0.));
#16845=DIRECTION('',(-0.857167300702115,-0.515038074910049,-1.04972719113862E-16));
#16846=DIRECTION('center_axis',(0.,-1.,0.));
#16847=DIRECTION('ref_axis',(1.,0.,0.));
#16848=DIRECTION('',(-0.85716730070211,-0.515038074910058,-1.04972719113862E-16));
#16849=DIRECTION('center_axis',(0.,-1.,0.));
#16850=DIRECTION('ref_axis',(1.,0.,0.));
#16851=DIRECTION('',(-0.85716730070211,-0.515038074910058,-1.04972719113862E-16));
#16852=DIRECTION('center_axis',(0.,-1.,0.));
#16853=DIRECTION('ref_axis',(1.,0.,0.));
#16854=DIRECTION('',(-0.85716730070211,-0.515038074910058,-1.04972719113862E-16));
#16855=DIRECTION('center_axis',(0.,-1.,0.));
#16856=DIRECTION('ref_axis',(1.,0.,0.));
#16857=DIRECTION('',(-0.85716730070211,-0.515038074910058,-1.04972719113862E-16));
#16858=DIRECTION('center_axis',(0.707106781186541,0.,-0.707106781186554));
#16859=DIRECTION('ref_axis',(-0.707106781186554,0.,-0.707106781186541));
#16860=DIRECTION('',(0.577350269189632,0.577350269189623,0.577350269189622));
#16861=DIRECTION('',(0.,-1.,0.));
#16862=DIRECTION('',(-0.577350269189632,-0.577350269189624,-0.577350269189622));
#16863=DIRECTION('',(-0.577350269189632,0.577350269189624,-0.577350269189622));
#16864=DIRECTION('',(0.,1.,0.));
#16865=DIRECTION('center_axis',(0.707106781186543,-0.707106781186552,0.));
#16866=DIRECTION('ref_axis',(0.,0.,-1.));
#16867=DIRECTION('',(0.,0.,1.));
#16868=DIRECTION('',(-0.577350269189628,-0.577350269189621,0.577350269189628));
#16869=DIRECTION('',(-0.577350269189628,-0.577350269189621,-0.577350269189628));
#16870=DIRECTION('',(0.577350269189632,0.577350269189624,-0.577350269189622));
#16871=DIRECTION('center_axis',(1.,0.,0.));
#16872=DIRECTION('ref_axis',(0.,0.,-1.));
#16873=DIRECTION('',(0.,0.,1.));
#16874=DIRECTION('',(0.,-1.,0.));
#16875=DIRECTION('',(0.,0.,1.));
#16876=DIRECTION('',(0.,1.,0.));
#16877=DIRECTION('',(0.,-0.707106781186553,-0.707106781186542));
#16878=DIRECTION('',(0.,0.,1.));
#16879=DIRECTION('',(0.,0.707106781186542,-0.707106781186553));
#16880=DIRECTION('',(0.,0.,1.));
#16881=DIRECTION('',(0.,-0.707106781186542,-0.707106781186553));
#16882=DIRECTION('',(0.,0.,1.));
#16883=DIRECTION('',(0.,0.707106781186542,-0.707106781186553));
#16884=DIRECTION('',(0.,-1.,0.));
#16885=DIRECTION('',(0.,0.,1.));
#16886=DIRECTION('',(0.,1.,0.));
#16887=DIRECTION('',(0.,0.,1.));
#16888=DIRECTION('',(0.,1.,0.));
#16889=DIRECTION('center_axis',(0.,0.707106781186547,-0.707106781186548));
#16890=DIRECTION('ref_axis',(-1.,0.,0.));
#16891=DIRECTION('',(-1.,0.,0.));
#16892=DIRECTION('',(0.577350269189627,-0.577350269189626,-0.577350269189625));
#16893=DIRECTION('',(1.,0.,0.));
#16894=DIRECTION('center_axis',(0.,-0.707106781186552,0.707106781186543));
#16895=DIRECTION('ref_axis',(1.,0.,0.));
#16896=DIRECTION('',(0.577350269189628,-0.577350269189621,-0.577350269189628));
#16897=DIRECTION('',(-1.,0.,0.));
#16898=DIRECTION('',(0.577350269189623,0.577350269189623,0.577350269189631));
#16899=DIRECTION('',(-0.577350269189623,0.577350269189624,0.577350269189631));
#16900=DIRECTION('center_axis',(0.707106781186548,0.,0.707106781186548));
#16901=DIRECTION('ref_axis',(0.707106781186548,0.,-0.707106781186548));
#16902=DIRECTION('',(-0.577350269189628,-0.577350269189621,0.577350269189628));
#16903=DIRECTION('',(0.,-1.,0.));
#16904=DIRECTION('center_axis',(0.,0.,1.));
#16905=DIRECTION('ref_axis',(0.,-1.,0.));
#16906=DIRECTION('',(1.,0.,0.));
#16907=DIRECTION('',(0.,1.,0.));
#16908=DIRECTION('center_axis',(-0.707106781186553,0.,0.707106781186543));
#16909=DIRECTION('ref_axis',(0.707106781186543,0.,0.707106781186553));
#16910=DIRECTION('',(-0.577350269189623,0.577350269189623,-0.577350269189631));
#16911=DIRECTION('',(0.,-1.,0.));
#16912=DIRECTION('',(0.577350269189623,-0.577350269189623,0.577350269189631));
#16913=DIRECTION('center_axis',(-0.707106781186548,-0.707106781186547,0.));
#16914=DIRECTION('ref_axis',(0.,0.,1.));
#16915=DIRECTION('',(0.,0.,-1.));
#16916=DIRECTION('',(0.577350269189626,-0.577350269189627,-0.577350269189624));
#16917=DIRECTION('',(0.577350269189626,-0.577350269189627,0.577350269189625));
#16918=DIRECTION('center_axis',(0.,-0.707106781186546,-0.707106781186549));
#16919=DIRECTION('ref_axis',(-1.,0.,0.));
#16920=DIRECTION('',(-0.577350269189627,-0.577350269189627,0.577350269189624));
#16921=DIRECTION('',(1.,0.,0.));
#16922=DIRECTION('center_axis',(-0.707106781186546,0.,-0.707106781186549));
#16923=DIRECTION('ref_axis',(-0.707106781186549,0.,0.707106781186546));
#16924=DIRECTION('',(0.,1.,0.));
#16925=DIRECTION('',(0.,-1.,0.));
#16926=DIRECTION('center_axis',(1.,0.,0.));
#16927=DIRECTION('ref_axis',(0.,0.,-1.));
#16928=DIRECTION('',(0.,0.,-1.));
#16929=DIRECTION('',(0.,-1.,0.));
#16930=DIRECTION('',(0.,0.,-1.));
#16931=DIRECTION('',(0.,1.,0.));
#16932=DIRECTION('',(0.,-0.707106781186542,0.707106781186553));
#16933=DIRECTION('',(0.,0.,-1.));
#16934=DIRECTION('',(0.,0.707106781186542,0.707106781186553));
#16935=DIRECTION('',(0.,0.,-1.));
#16936=DIRECTION('',(0.,-0.707106781186542,0.707106781186553));
#16937=DIRECTION('',(0.,0.,-1.));
#16938=DIRECTION('',(0.,0.707106781186553,0.707106781186542));
#16939=DIRECTION('',(0.,-1.,0.));
#16940=DIRECTION('',(0.,0.,-1.));
#16941=DIRECTION('',(0.,1.,0.));
#16942=DIRECTION('',(0.,0.,-1.));
#16943=DIRECTION('center_axis',(0.,0.707106781186542,-0.707106781186553));
#16944=DIRECTION('ref_axis',(-1.,0.,0.));
#16945=DIRECTION('',(-1.,0.,0.));
#16946=DIRECTION('',(1.,0.,0.));
#16947=DIRECTION('center_axis',(0.,1.,0.));
#16948=DIRECTION('ref_axis',(0.,0.,1.));
#16949=DIRECTION('',(-1.,0.,0.));
#16950=DIRECTION('center_axis',(0.,0.707106781186553,0.707106781186542));
#16951=DIRECTION('ref_axis',(1.,0.,0.));
#16952=DIRECTION('center_axis',(0.,0.707106781186553,-0.707106781186542));
#16953=DIRECTION('ref_axis',(-1.,0.,0.));
#16954=DIRECTION('',(1.,0.,0.));
#16955=DIRECTION('center_axis',(0.,1.,0.));
#16956=DIRECTION('ref_axis',(0.,0.,1.));
#16957=DIRECTION('',(-1.,0.,0.));
#16958=DIRECTION('center_axis',(0.,0.707106781186553,0.707106781186542));
#16959=DIRECTION('ref_axis',(1.,0.,0.));
#16960=DIRECTION('',(1.,0.,0.));
#16961=DIRECTION('center_axis',(0.,0.,1.));
#16962=DIRECTION('ref_axis',(0.,-1.,0.));
#16963=DIRECTION('',(1.,0.,0.));
#16964=DIRECTION('center_axis',(0.,0.707106781186552,0.707106781186543));
#16965=DIRECTION('ref_axis',(1.,0.,0.));
#16966=DIRECTION('',(-1.,0.,0.));
#16967=DIRECTION('center_axis',(0.,1.,0.));
#16968=DIRECTION('ref_axis',(0.,0.,1.));
#16969=DIRECTION('',(1.,0.,0.));
#16970=DIRECTION('center_axis',(0.,0.,-1.));
#16971=DIRECTION('ref_axis',(0.,1.,0.));
#16972=DIRECTION('center_axis',(0.,1.,0.));
#16973=DIRECTION('ref_axis',(0.,0.,1.));
#16974=DIRECTION('',(1.,0.,0.));
#16975=DIRECTION('center_axis',(0.,0.,-1.));
#16976=DIRECTION('ref_axis',(0.,1.,0.));
#16977=DIRECTION('',(1.,0.,0.));
#16978=DIRECTION('center_axis',(0.,1.,0.));
#16979=DIRECTION('ref_axis',(0.,0.,1.));
#16980=DIRECTION('center_axis',(0.,1.,0.));
#16981=DIRECTION('ref_axis',(0.,0.,1.));
#16982=DIRECTION('center_axis',(0.,0.,-1.));
#16983=DIRECTION('ref_axis',(0.,1.,0.));
#16984=DIRECTION('',(1.,0.,0.));
#16985=DIRECTION('center_axis',(0.,1.,0.));
#16986=DIRECTION('ref_axis',(0.,0.,1.));
#16987=DIRECTION('',(1.,0.,0.));
#16988=DIRECTION('center_axis',(0.,0.,1.));
#16989=DIRECTION('ref_axis',(0.,-1.,0.));
#20563=CARTESIAN_POINT('',(0.,0.,0.));
#20564=CARTESIAN_POINT('Origin',(180.,21.,55.65));
#20565=CARTESIAN_POINT('',(177.25,21.,55.8));
#20566=CARTESIAN_POINT('Origin',(180.,21.,55.8));
#20567=CARTESIAN_POINT('',(176.95,21.,55.5));
#20568=CARTESIAN_POINT('',(177.1,21.,55.65));
#20569=CARTESIAN_POINT('Origin',(180.,21.,55.5));
#20570=CARTESIAN_POINT('Origin',(0.,13.,55.5));
#20571=CARTESIAN_POINT('',(210.,31.2,55.5));
#20572=CARTESIAN_POINT('',(0.,31.2,55.5));
#20573=CARTESIAN_POINT('',(0.,31.2,55.5));
#20574=CARTESIAN_POINT('',(210.,13.,55.5));
#20575=CARTESIAN_POINT('',(210.,31.5,55.5));
#20576=CARTESIAN_POINT('',(0.,13.,55.5));
#20577=CARTESIAN_POINT('',(0.,13.,55.5));
#20578=CARTESIAN_POINT('',(0.,31.5,55.5));
#20579=CARTESIAN_POINT('',(26.95,21.,55.5));
#20580=CARTESIAN_POINT('Origin',(30.,21.,55.5));
#20581=CARTESIAN_POINT('',(126.95,21.,55.5));
#20582=CARTESIAN_POINT('Origin',(130.,21.,55.5));
#20583=CARTESIAN_POINT('',(76.95,21.,55.5));
#20584=CARTESIAN_POINT('Origin',(80.,21.,55.5));
#20585=CARTESIAN_POINT('Origin',(180.,21.,55.5));
#20586=CARTESIAN_POINT('',(177.25,21.,60.5));
#20587=CARTESIAN_POINT('',(177.25,21.,55.5));
#20588=CARTESIAN_POINT('Origin',(180.,21.,60.5));
#20589=CARTESIAN_POINT('Origin',(30.,21.,55.65));
#20590=CARTESIAN_POINT('',(27.25,21.,55.8));
#20591=CARTESIAN_POINT('Origin',(30.,21.,55.8));
#20592=CARTESIAN_POINT('',(27.1,21.,55.65));
#20593=CARTESIAN_POINT('Origin',(30.,21.,55.5));
#20594=CARTESIAN_POINT('',(27.25,21.,60.5));
#20595=CARTESIAN_POINT('',(27.25,21.,55.5));
#20596=CARTESIAN_POINT('Origin',(30.,21.,60.5));
#20597=CARTESIAN_POINT('Origin',(80.,21.,55.65));
#20598=CARTESIAN_POINT('',(77.25,21.,55.8));
#20599=CARTESIAN_POINT('Origin',(80.,21.,55.8));
#20600=CARTESIAN_POINT('',(77.1,21.,55.65));
#20601=CARTESIAN_POINT('Origin',(80.,21.,55.5));
#20602=CARTESIAN_POINT('',(77.25,21.,60.5));
#20603=CARTESIAN_POINT('',(77.25,21.,55.5));
#20604=CARTESIAN_POINT('Origin',(80.,21.,60.5));
#20605=CARTESIAN_POINT('Origin',(130.,21.,55.65));
#20606=CARTESIAN_POINT('',(127.25,21.,55.8));
#20607=CARTESIAN_POINT('Origin',(130.,21.,55.8));
#20608=CARTESIAN_POINT('',(127.1,21.,55.65));
#20609=CARTESIAN_POINT('Origin',(130.,21.,55.5));
#20610=CARTESIAN_POINT('',(127.25,21.,60.5));
#20611=CARTESIAN_POINT('',(127.25,21.,55.5));
#20612=CARTESIAN_POINT('Origin',(130.,21.,60.5));
#20613=CARTESIAN_POINT('Origin',(180.,21.,44.35));
#20614=CARTESIAN_POINT('',(177.25,21.,44.2));
#20615=CARTESIAN_POINT('Origin',(180.,21.,44.2));
#20616=CARTESIAN_POINT('',(176.95,21.,44.5));
#20617=CARTESIAN_POINT('',(177.1,21.,44.35));
#20618=CARTESIAN_POINT('Origin',(180.,21.,44.5));
#20619=CARTESIAN_POINT('Origin',(0.,31.5,44.5));
#20620=CARTESIAN_POINT('',(0.,31.2,44.5));
#20621=CARTESIAN_POINT('',(210.,31.2,44.5));
#20622=CARTESIAN_POINT('',(0.,31.2,44.5));
#20623=CARTESIAN_POINT('',(0.,13.,44.5));
#20624=CARTESIAN_POINT('',(0.,13.,44.5));
#20625=CARTESIAN_POINT('',(210.,13.,44.5));
#20626=CARTESIAN_POINT('',(0.,13.,44.5));
#20627=CARTESIAN_POINT('',(210.,13.,44.5));
#20628=CARTESIAN_POINT('',(26.95,21.,44.5));
#20629=CARTESIAN_POINT('Origin',(30.,21.,44.5));
#20630=CARTESIAN_POINT('',(126.95,21.,44.5));
#20631=CARTESIAN_POINT('Origin',(130.,21.,44.5));
#20632=CARTESIAN_POINT('',(76.95,21.,44.5));
#20633=CARTESIAN_POINT('Origin',(80.,21.,44.5));
#20634=CARTESIAN_POINT('Origin',(180.,21.,44.5));
#20635=CARTESIAN_POINT('',(177.25,21.,39.5));
#20636=CARTESIAN_POINT('',(177.25,21.,44.5));
#20637=CARTESIAN_POINT('Origin',(180.,21.,39.5));
#20638=CARTESIAN_POINT('Origin',(30.,21.,44.35));
#20639=CARTESIAN_POINT('',(27.25,21.,44.2));
#20640=CARTESIAN_POINT('Origin',(30.,21.,44.2));
#20641=CARTESIAN_POINT('',(27.1,21.,44.35));
#20642=CARTESIAN_POINT('Origin',(30.,21.,44.5));
#20643=CARTESIAN_POINT('',(27.25,21.,39.5));
#20644=CARTESIAN_POINT('',(27.25,21.,44.5));
#20645=CARTESIAN_POINT('Origin',(30.,21.,39.5));
#20646=CARTESIAN_POINT('Origin',(80.,21.,44.35));
#20647=CARTESIAN_POINT('',(77.25,21.,44.2));
#20648=CARTESIAN_POINT('Origin',(80.,21.,44.2));
#20649=CARTESIAN_POINT('',(77.1,21.,44.35));
#20650=CARTESIAN_POINT('Origin',(80.,21.,44.5));
#20651=CARTESIAN_POINT('',(77.25,21.,39.5));
#20652=CARTESIAN_POINT('',(77.25,21.,44.5));
#20653=CARTESIAN_POINT('Origin',(80.,21.,39.5));
#20654=CARTESIAN_POINT('Origin',(130.,21.,44.35));
#20655=CARTESIAN_POINT('',(127.25,21.,44.2));
#20656=CARTESIAN_POINT('Origin',(130.,21.,44.2));
#20657=CARTESIAN_POINT('',(127.1,21.,44.35));
#20658=CARTESIAN_POINT('Origin',(130.,21.,44.5));
#20659=CARTESIAN_POINT('',(127.25,21.,39.5));
#20660=CARTESIAN_POINT('',(127.25,21.,44.5));
#20661=CARTESIAN_POINT('Origin',(130.,21.,39.5));
#20662=CARTESIAN_POINT('Origin',(200.,0.2,80.));
#20663=CARTESIAN_POINT('',(196.95,0.4,80.));
#20664=CARTESIAN_POINT('Origin',(200.,0.4,80.));
#20665=CARTESIAN_POINT('',(196.55,0.,80.));
#20666=CARTESIAN_POINT('',(196.75,0.2,80.));
#20667=CARTESIAN_POINT('Origin',(200.,0.,80.));
#20668=CARTESIAN_POINT('Origin',(0.,0.,100.));
#20669=CARTESIAN_POINT('',(209.5,0.,99.5));
#20670=CARTESIAN_POINT('',(209.5,0.,0.499999999999998));
#20671=CARTESIAN_POINT('',(209.5,0.,75.));
#20672=CARTESIAN_POINT('',(0.5,0.,99.5));
#20673=CARTESIAN_POINT('',(0.,0.,99.5));
#20674=CARTESIAN_POINT('',(0.5,0.,0.499999999999998));
#20675=CARTESIAN_POINT('',(0.5,0.,75.));
#20676=CARTESIAN_POINT('',(0.,0.,0.499999999999998));
#20677=CARTESIAN_POINT('',(146.55,0.,80.));
#20678=CARTESIAN_POINT('Origin',(150.,0.,80.));
#20679=CARTESIAN_POINT('',(56.55,0.,20.));
#20680=CARTESIAN_POINT('Origin',(60.,0.,20.));
#20681=CARTESIAN_POINT('',(56.55,0.,80.));
#20682=CARTESIAN_POINT('Origin',(60.,0.,80.));
#20683=CARTESIAN_POINT('',(196.55,0.,20.));
#20684=CARTESIAN_POINT('Origin',(200.,0.,20.));
#20685=CARTESIAN_POINT('',(146.55,0.,20.));
#20686=CARTESIAN_POINT('Origin',(150.,0.,20.));
#20687=CARTESIAN_POINT('',(6.55,0.,80.));
#20688=CARTESIAN_POINT('Origin',(10.,0.,80.));
#20689=CARTESIAN_POINT('',(6.55,0.,20.));
#20690=CARTESIAN_POINT('Origin',(10.,0.,20.));
#20691=CARTESIAN_POINT('Origin',(200.,0.,80.));
#20692=CARTESIAN_POINT('',(196.95,8.,80.));
#20693=CARTESIAN_POINT('',(196.95,0.,80.));
#20694=CARTESIAN_POINT('Origin',(200.,8.,80.));
#20695=CARTESIAN_POINT('Origin',(150.,0.2,80.));
#20696=CARTESIAN_POINT('',(146.95,0.4,80.));
#20697=CARTESIAN_POINT('Origin',(150.,0.4,80.));
#20698=CARTESIAN_POINT('',(146.75,0.2,80.));
#20699=CARTESIAN_POINT('Origin',(150.,0.,80.));
#20700=CARTESIAN_POINT('',(146.95,8.,80.));
#20701=CARTESIAN_POINT('',(146.95,0.,80.));
#20702=CARTESIAN_POINT('Origin',(150.,8.,80.));
#20703=CARTESIAN_POINT('Origin',(10.,0.2,20.));
#20704=CARTESIAN_POINT('',(6.95,0.4,20.));
#20705=CARTESIAN_POINT('Origin',(10.,0.4,20.));
#20706=CARTESIAN_POINT('',(6.75,0.2,20.));
#20707=CARTESIAN_POINT('Origin',(10.,0.,20.));
#20708=CARTESIAN_POINT('',(6.95,8.,20.));
#20709=CARTESIAN_POINT('',(6.95,0.,20.));
#20710=CARTESIAN_POINT('Origin',(10.,8.,20.));
#20711=CARTESIAN_POINT('Origin',(60.,0.2,20.));
#20712=CARTESIAN_POINT('',(56.95,0.4,20.));
#20713=CARTESIAN_POINT('Origin',(60.,0.4,20.));
#20714=CARTESIAN_POINT('',(56.75,0.2,20.));
#20715=CARTESIAN_POINT('Origin',(60.,0.,20.));
#20716=CARTESIAN_POINT('',(56.95,8.,20.));
#20717=CARTESIAN_POINT('',(56.95,0.,20.));
#20718=CARTESIAN_POINT('Origin',(60.,8.,20.));
#20719=CARTESIAN_POINT('Origin',(10.,0.2,80.));
#20720=CARTESIAN_POINT('',(6.95,0.4,80.));
#20721=CARTESIAN_POINT('Origin',(10.,0.4,80.));
#20722=CARTESIAN_POINT('',(6.75,0.2,80.));
#20723=CARTESIAN_POINT('Origin',(10.,0.,80.));
#20724=CARTESIAN_POINT('',(6.95,8.,80.));
#20725=CARTESIAN_POINT('',(6.95,0.,80.));
#20726=CARTESIAN_POINT('Origin',(10.,8.,80.));
#20727=CARTESIAN_POINT('Origin',(60.,0.2,80.));
#20728=CARTESIAN_POINT('',(56.95,0.4,80.));
#20729=CARTESIAN_POINT('Origin',(60.,0.4,80.));
#20730=CARTESIAN_POINT('',(56.75,0.2,80.));
#20731=CARTESIAN_POINT('Origin',(60.,0.,80.));
#20732=CARTESIAN_POINT('',(56.95,8.,80.));
#20733=CARTESIAN_POINT('',(56.95,0.,80.));
#20734=CARTESIAN_POINT('Origin',(60.,8.,80.));
#20735=CARTESIAN_POINT('Origin',(150.,0.2,20.));
#20736=CARTESIAN_POINT('',(146.95,0.4,20.));
#20737=CARTESIAN_POINT('Origin',(150.,0.4,20.));
#20738=CARTESIAN_POINT('',(146.75,0.2,20.));
#20739=CARTESIAN_POINT('Origin',(150.,0.,20.));
#20740=CARTESIAN_POINT('',(146.95,8.,20.));
#20741=CARTESIAN_POINT('',(146.95,0.,20.));
#20742=CARTESIAN_POINT('Origin',(150.,8.,20.));
#20743=CARTESIAN_POINT('Origin',(200.,0.2,20.));
#20744=CARTESIAN_POINT('',(196.95,0.4,20.));
#20745=CARTESIAN_POINT('Origin',(200.,0.4,20.));
#20746=CARTESIAN_POINT('',(196.75,0.2,20.));
#20747=CARTESIAN_POINT('Origin',(200.,0.,20.));
#20748=CARTESIAN_POINT('',(196.95,8.,20.));
#20749=CARTESIAN_POINT('',(196.95,0.,20.));
#20750=CARTESIAN_POINT('Origin',(200.,8.,20.));
#20751=CARTESIAN_POINT('Origin',(200.,8.91631244401703,80.));
#20752=CARTESIAN_POINT('',(200.,9.83262488803406,80.));
#20753=CARTESIAN_POINT('',(198.475,8.91631244401703,80.));
#20754=CARTESIAN_POINT('Origin',(200.,8.91631244401703,20.));
#20755=CARTESIAN_POINT('',(200.,9.83262488803406,20.));
#20756=CARTESIAN_POINT('',(198.475,8.91631244401703,20.));
#20757=CARTESIAN_POINT('Origin',(150.,8.91631244401703,80.));
#20758=CARTESIAN_POINT('',(150.,9.83262488803406,80.));
#20759=CARTESIAN_POINT('',(148.475,8.91631244401703,80.));
#20760=CARTESIAN_POINT('Origin',(150.,8.91631244401703,20.));
#20761=CARTESIAN_POINT('',(150.,9.83262488803406,20.));
#20762=CARTESIAN_POINT('',(148.475,8.91631244401703,20.));
#20763=CARTESIAN_POINT('Origin',(60.,8.91631244401703,80.));
#20764=CARTESIAN_POINT('',(60.,9.83262488803406,80.));
#20765=CARTESIAN_POINT('',(58.475,8.91631244401703,80.));
#20766=CARTESIAN_POINT('Origin',(60.,8.91631244401703,20.));
#20767=CARTESIAN_POINT('',(60.,9.83262488803406,20.));
#20768=CARTESIAN_POINT('',(58.475,8.91631244401703,20.));
#20769=CARTESIAN_POINT('Origin',(10.,8.91631244401703,80.));
#20770=CARTESIAN_POINT('',(10.,9.83262488803406,80.));
#20771=CARTESIAN_POINT('',(8.475,8.91631244401703,80.));
#20772=CARTESIAN_POINT('Origin',(10.,8.91631244401703,20.));
#20773=CARTESIAN_POINT('',(10.,9.83262488803406,20.));
#20774=CARTESIAN_POINT('',(8.475,8.91631244401703,20.));
#20775=CARTESIAN_POINT('Origin',(209.75,7.875,0.249999999999999));
#20776=CARTESIAN_POINT('',(209.5,12.5,0.));
#20777=CARTESIAN_POINT('',(210.,13.,0.499999999999998));
#20778=CARTESIAN_POINT('',(173.979166666666,-23.0208333333335,-35.5208333333335));
#20779=CARTESIAN_POINT('',(210.,0.5,0.499999999999998));
#20780=CARTESIAN_POINT('',(210.,7.875,0.499999999999998));
#20781=CARTESIAN_POINT('',(209.75,0.250000000000012,0.249999999999995));
#20782=CARTESIAN_POINT('',(223.479166666667,13.9791666666665,13.9791666666665));
#20783=CARTESIAN_POINT('',(209.5,0.5,0.));
#20784=CARTESIAN_POINT('',(173.520833333333,36.4791666666669,-35.9791666666668));
#20785=CARTESIAN_POINT('',(209.5,7.875,0.));
#20786=CARTESIAN_POINT('Origin',(209.75,0.25,75.));
#20787=CARTESIAN_POINT('',(210.,0.5,99.5));
#20788=CARTESIAN_POINT('',(210.,0.5,75.));
#20789=CARTESIAN_POINT('',(209.75,0.249999999999986,99.75));
#20790=CARTESIAN_POINT('',(216.229166666667,6.72916666666661,93.2708333333333));
#20791=CARTESIAN_POINT('',(170.666666666666,-38.8333333333332,60.6666666666663));
#20792=CARTESIAN_POINT('',(162.333333333333,-47.1666666666668,47.6666666666666));
#20793=CARTESIAN_POINT('Origin',(210.,15.75,50.));
#20794=CARTESIAN_POINT('',(210.,13.,24.));
#20795=CARTESIAN_POINT('',(210.,13.,24.));
#20796=CARTESIAN_POINT('',(210.,5.5,24.));
#20797=CARTESIAN_POINT('',(210.,5.5,24.));
#20798=CARTESIAN_POINT('',(210.,5.5,39.5));
#20799=CARTESIAN_POINT('',(210.,5.5,39.5));
#20800=CARTESIAN_POINT('',(210.,31.2,39.5));
#20801=CARTESIAN_POINT('',(210.,31.5,39.5));
#20802=CARTESIAN_POINT('',(210.,31.5,39.8));
#20803=CARTESIAN_POINT('',(210.,30.0374999999999,38.3375));
#20804=CARTESIAN_POINT('',(210.,31.5,44.2));
#20805=CARTESIAN_POINT('',(210.,31.5,44.5));
#20806=CARTESIAN_POINT('',(210.,26.0375000000001,49.6625));
#20807=CARTESIAN_POINT('',(210.,13.,55.5));
#20808=CARTESIAN_POINT('',(210.,31.5,55.8));
#20809=CARTESIAN_POINT('',(210.,26.0375000000001,50.3375));
#20810=CARTESIAN_POINT('',(210.,31.5,60.2));
#20811=CARTESIAN_POINT('',(210.,31.5,60.5));
#20812=CARTESIAN_POINT('',(210.,31.2,60.5));
#20813=CARTESIAN_POINT('',(210.,30.0375000000001,61.6625));
#20814=CARTESIAN_POINT('',(210.,5.5,60.5));
#20815=CARTESIAN_POINT('',(210.,5.5,60.5));
#20816=CARTESIAN_POINT('',(210.,5.5,76.));
#20817=CARTESIAN_POINT('',(210.,5.5,76.));
#20818=CARTESIAN_POINT('',(210.,13.,76.));
#20819=CARTESIAN_POINT('',(210.,13.,76.));
#20820=CARTESIAN_POINT('',(210.,13.,99.5));
#20821=CARTESIAN_POINT('',(210.,13.,100.));
#20822=CARTESIAN_POINT('',(210.,14.375,99.5));
#20823=CARTESIAN_POINT('Origin',(0.,12.75,0.25));
#20824=CARTESIAN_POINT('',(0.5,12.5,0.));
#20825=CARTESIAN_POINT('',(0.,12.5,0.));
#20826=CARTESIAN_POINT('',(0.,13.,0.499999999999998));
#20827=CARTESIAN_POINT('',(1.02083333333333,11.9791666666667,-0.520833333333332));
#20828=CARTESIAN_POINT('',(0.,13.,0.5));
#20829=CARTESIAN_POINT('Origin',(0.,0.25,99.75));
#20830=CARTESIAN_POINT('',(209.5,0.5,100.));
#20831=CARTESIAN_POINT('',(172.4375,37.5624999999998,137.0625));
#20832=CARTESIAN_POINT('',(0.5,0.5,100.));
#20833=CARTESIAN_POINT('',(0.,0.5,100.));
#20834=CARTESIAN_POINT('',(0.25,0.250000000000001,99.75));
#20835=CARTESIAN_POINT('',(2.56249999999998,2.56249999999998,102.0625));
#20836=CARTESIAN_POINT('',(4.33333333333335,-3.83333333333335,95.6666666666666));
#20837=CARTESIAN_POINT('Origin',(209.75,14.375,99.75));
#20838=CARTESIAN_POINT('',(209.5,12.5,100.));
#20839=CARTESIAN_POINT('',(175.0625,-21.9374999999999,134.4375));
#20840=CARTESIAN_POINT('',(209.5,14.375,100.));
#20841=CARTESIAN_POINT('Origin',(0.,13.,100.));
#20842=CARTESIAN_POINT('',(0.5,12.5,100.));
#20843=CARTESIAN_POINT('',(0.,12.5,100.));
#20844=CARTESIAN_POINT('',(0.5,14.375,100.));
#20845=CARTESIAN_POINT('Origin',(0.25,14.375,99.75));
#20846=CARTESIAN_POINT('',(0.,13.,99.5));
#20847=CARTESIAN_POINT('',(-0.0624999999999985,13.0625,99.4375));
#20848=CARTESIAN_POINT('',(0.,0.5,99.5));
#20849=CARTESIAN_POINT('',(0.,14.375,99.5));
#20850=CARTESIAN_POINT('',(-6.22916666666666,6.72916666666667,93.2708333333333));
#20851=CARTESIAN_POINT('Origin',(0.25,0.25,75.));
#20852=CARTESIAN_POINT('',(0.,0.5,0.499999999999998));
#20853=CARTESIAN_POINT('',(0.,0.5,75.));
#20854=CARTESIAN_POINT('',(0.25,0.25,0.25));
#20855=CARTESIAN_POINT('',(-13.4791666666666,13.9791666666667,13.9791666666666));
#20856=CARTESIAN_POINT('',(12.6666666666666,-12.1666666666667,12.6666666666666));
#20857=CARTESIAN_POINT('Origin',(0.,0.25,0.249999999999999));
#20858=CARTESIAN_POINT('',(0.5,0.5,0.));
#20859=CARTESIAN_POINT('',(1.47916666666667,1.47916666666667,-0.979166666666666));
#20860=CARTESIAN_POINT('',(0.,0.5,0.));
#20861=CARTESIAN_POINT('Origin',(0.25,7.875,0.249999999999999));
#20862=CARTESIAN_POINT('',(0.,7.875,0.499999999999998));
#20863=CARTESIAN_POINT('',(0.5,7.875,0.));
#20864=CARTESIAN_POINT('Origin',(0.,15.75,50.));
#20865=CARTESIAN_POINT('',(0.,13.,76.));
#20866=CARTESIAN_POINT('',(0.,13.,100.));
#20867=CARTESIAN_POINT('',(0.,5.5,76.));
#20868=CARTESIAN_POINT('',(0.,13.,76.));
#20869=CARTESIAN_POINT('',(0.,5.5,60.5));
#20870=CARTESIAN_POINT('',(0.,5.5,76.));
#20871=CARTESIAN_POINT('',(0.,31.2,60.5));
#20872=CARTESIAN_POINT('',(0.,5.5,60.5));
#20873=CARTESIAN_POINT('',(0.,31.5,60.2));
#20874=CARTESIAN_POINT('',(0.,30.0375000000001,61.6625));
#20875=CARTESIAN_POINT('',(0.,31.5,55.8));
#20876=CARTESIAN_POINT('',(0.,31.5,60.5));
#20877=CARTESIAN_POINT('',(0.,26.0375000000001,50.3375));
#20878=CARTESIAN_POINT('',(0.,13.,55.5));
#20879=CARTESIAN_POINT('',(0.,31.5,44.2));
#20880=CARTESIAN_POINT('',(0.,26.0375000000001,49.6625));
#20881=CARTESIAN_POINT('',(0.,31.5,39.8));
#20882=CARTESIAN_POINT('',(0.,31.5,44.5));
#20883=CARTESIAN_POINT('',(0.,31.2,39.5));
#20884=CARTESIAN_POINT('',(0.,30.0374999999999,38.3375));
#20885=CARTESIAN_POINT('',(0.,5.5,39.5));
#20886=CARTESIAN_POINT('',(0.,31.5,39.5));
#20887=CARTESIAN_POINT('',(0.,5.5,24.));
#20888=CARTESIAN_POINT('',(0.,5.5,39.5));
#20889=CARTESIAN_POINT('',(0.,13.,24.));
#20890=CARTESIAN_POINT('',(0.,5.5,24.));
#20891=CARTESIAN_POINT('',(0.,13.,24.));
#20892=CARTESIAN_POINT('Origin',(0.,31.35,39.65));
#20893=CARTESIAN_POINT('',(0.,31.2,39.5));
#20894=CARTESIAN_POINT('',(0.,31.5,39.8));
#20895=CARTESIAN_POINT('Origin',(0.,31.5,39.5));
#20896=CARTESIAN_POINT('',(0.,31.5,44.2));
#20897=CARTESIAN_POINT('Origin',(0.,31.35,44.35));
#20898=CARTESIAN_POINT('Origin',(0.,31.35,55.65));
#20899=CARTESIAN_POINT('',(0.,31.5,55.8));
#20900=CARTESIAN_POINT('Origin',(0.,31.5,55.5));
#20901=CARTESIAN_POINT('',(0.,31.5,60.2));
#20902=CARTESIAN_POINT('Origin',(0.,31.35,60.35));
#20903=CARTESIAN_POINT('',(0.,31.2,60.5));
#20904=CARTESIAN_POINT('Origin',(0.,31.5,60.5));
#20905=CARTESIAN_POINT('',(0.,5.5,60.5));
#20906=CARTESIAN_POINT('Origin',(0.,12.75,99.75));
#20907=CARTESIAN_POINT('',(0.,13.,99.5));
#20908=CARTESIAN_POINT('Origin',(0.,13.,0.));
#20909=CARTESIAN_POINT('',(0.,13.,24.));
#20910=CARTESIAN_POINT('Origin',(0.,0.,0.));
#20911=CARTESIAN_POINT('Origin',(0.,13.,76.));
#20912=CARTESIAN_POINT('',(0.,13.,76.));
#20913=CARTESIAN_POINT('Origin',(0.,5.5,76.));
#20914=CARTESIAN_POINT('',(0.,5.5,76.));
#20915=CARTESIAN_POINT('Origin',(0.,5.5,60.5));
#20916=CARTESIAN_POINT('Origin',(0.,13.,44.5));
#20917=CARTESIAN_POINT('Origin',(0.,5.5,39.5));
#20918=CARTESIAN_POINT('',(0.,5.5,39.5));
#20919=CARTESIAN_POINT('Origin',(0.,5.5,24.));
#20920=CARTESIAN_POINT('',(0.,5.5,24.));
#20921=CARTESIAN_POINT('Origin',(0.,13.,24.));
#81018=UNCERTAINTY_MEASURE_WITH_UNIT(LENGTH_MEASURE(0.01),#81041,
'DISTANCE_ACCURACY_VALUE',
'Maximum model space distance between geometric entities at asserted c
onnectivities');
#81028=UNCERTAINTY_MEASURE_WITH_UNIT(LENGTH_MEASURE(0.01),#81041,
'DISTANCE_ACCURACY_VALUE',
'Maximum model space distance between geometric entities at asserted c
onnectivities');
#81030=(
GEOMETRIC_REPRESENTATION_CONTEXT(3)
GLOBAL_UNCERTAINTY_ASSIGNED_CONTEXT((#81018))
GLOBAL_UNIT_ASSIGNED_CONTEXT((#81041,#81043,#81044))
REPRESENTATION_CONTEXT('','3D')
);
#81040=(
GEOMETRIC_REPRESENTATION_CONTEXT(3)
GLOBAL_UNCERTAINTY_ASSIGNED_CONTEXT((#81028))
GLOBAL_UNIT_ASSIGNED_CONTEXT((#81041,#81043,#81044))
REPRESENTATION_CONTEXT('','3D')
);
#81041=(
LENGTH_UNIT()
NAMED_UNIT(*)
SI_UNIT(.MILLI.,.METRE.)
);
#81043=(
NAMED_UNIT(*)
PLANE_ANGLE_UNIT()
SI_UNIT($,.RADIAN.)
);
#81044=(
NAMED_UNIT(*)
SI_UNIT($,.STERADIAN.)
SOLID_ANGLE_UNIT()
);
#81046=SHAPE_DEFINITION_REPRESENTATION(#81057,#81130);
#81057=PRODUCT_DEFINITION_SHAPE('',$,#81142);
#81130=SHAPE_REPRESENTATION('',(#15206),#81030);
#81140=PRODUCT_DEFINITION_CONTEXT('part definition',#81175,'design');
#81142=PRODUCT_DEFINITION('Base - Stationary Rail Block',
'Base - Stationary Rail Block',#81153,#81140);
#81153=PRODUCT_DEFINITION_FORMATION('',$,#81178);
#81175=APPLICATION_CONTEXT(
'Core Data for Automotive Mechanical Design Process');
#81176=PRODUCT_CONTEXT('part definition',#81175,'mechanical');
#81178=PRODUCT('Base - Stationary Rail Block',
'Base - Stationary Rail Block',$,(#81176));
#81189=PRESENTATION_STYLE_ASSIGNMENT((#81200));
#81200=SURFACE_STYLE_USAGE(.BOTH.,#81211);
#81211=SURFACE_SIDE_STYLE('',(#81222));
#81222=SURFACE_STYLE_FILL_AREA(#81233);
#81233=FILL_AREA_STYLE('Opaque(204,208,214)',(#81244));
#81244=FILL_AREA_STYLE_COLOUR('Opaque(204,208,214)',#81255);
#81255=COLOUR_RGB('Opaque(204,208,214)', 0.09019608, 0.27058824, 0.51372549);
ENDSEC;
END-ISO-10303-21;
